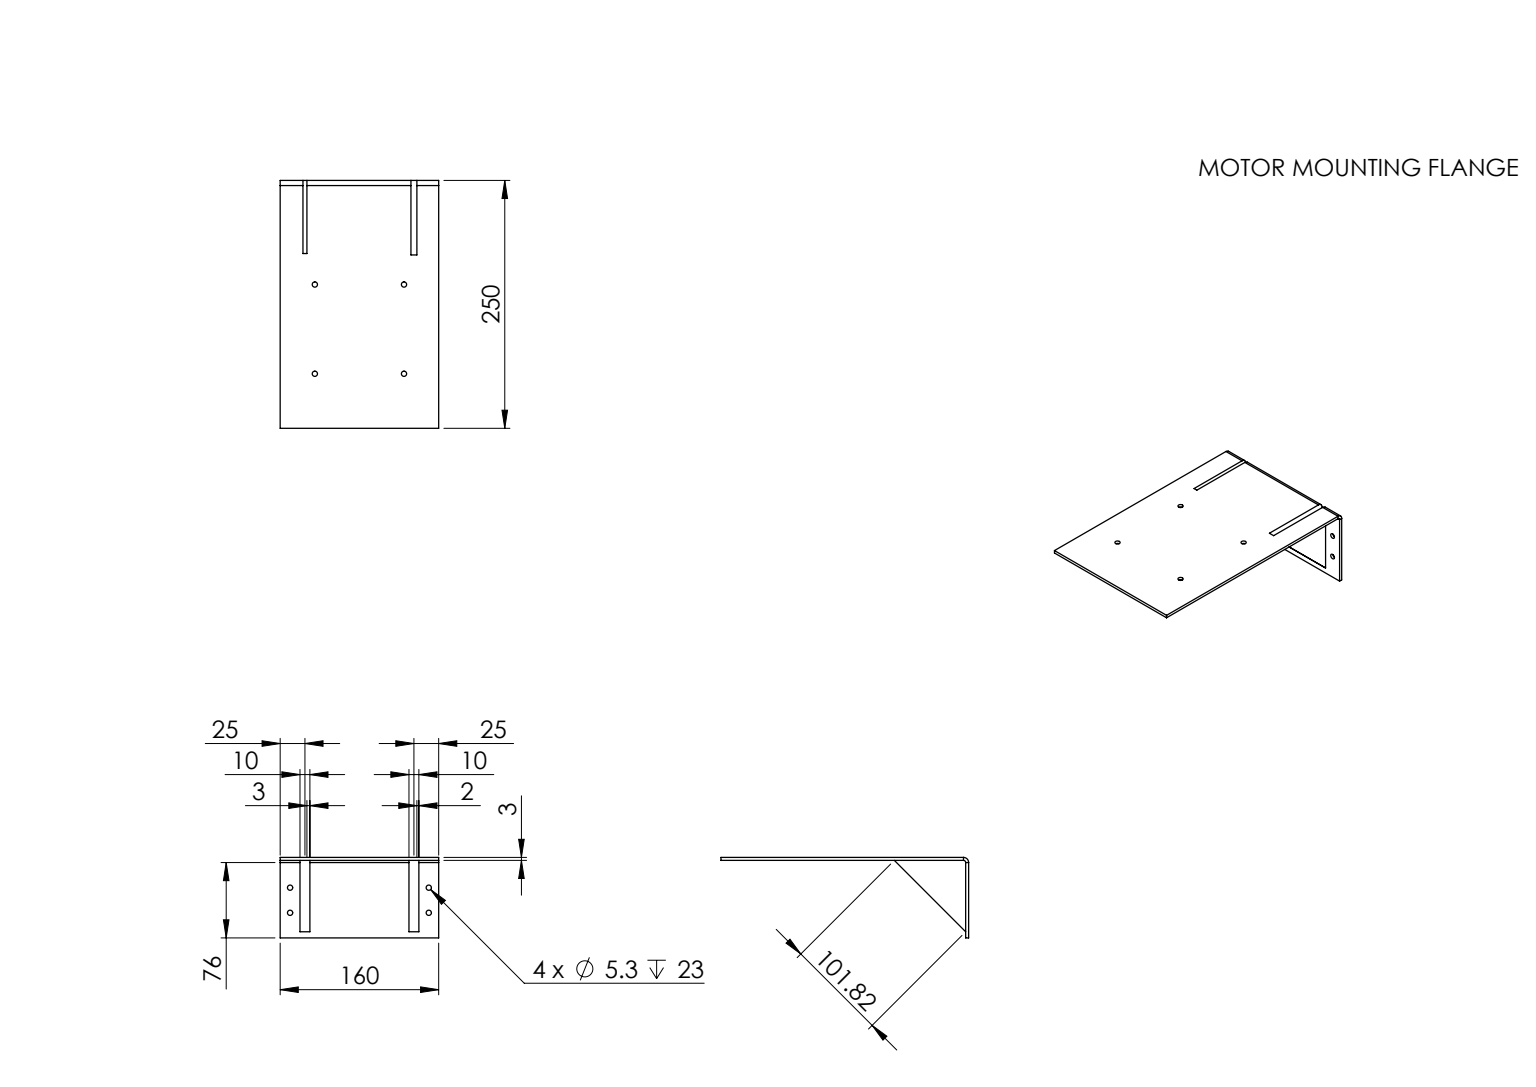
ISO-10303-21;
HEADER;
FILE_DESCRIPTION (('STEP AP214'),
    '1' );
FILE_NAME ('motor mounting flange.step',
    '2026-10-31T03:46:07',
    ( '' ),
    ( '' ),
    'SwSTEP 2.0',
    'SolidWorks 2026',
    '' );
FILE_SCHEMA (( 'AUTOMOTIVE_DESIGN' ));
ENDSEC;

DATA;
#7=VECTOR ( 'NONE', #7349, 1000.000000000000000 ) ;
#29=DIRECTION ( 'NONE',  ( 0.000000000000000000, 0.7071067811865489050, 0.7071067811865462405 ) ) ;
#48=CARTESIAN_POINT ( 'NONE',  ( 80.00000000000004263, -137.9999999999999716, 3.000000000000000000 ) ) ;
#90=EDGE_LOOP ( 'NONE', ( #21123, #7756, #684, #7867 ) ) ;
#122=DIRECTION ( 'NONE',  ( -1.000000000000000000, 3.051161311199799893E-31, 8.144298233840332611E-17 ) ) ;
#142=ORIENTED_EDGE ( 'NONE', *, *, #15816, .T. ) ;
#152=DIRECTION ( 'NONE',  ( 0.000000000000000000, 0.000000000000000000, -1.000000000000000000 ) ) ;
#157=EDGE_CURVE ( 'NONE', #8899, #17134, #9062, .T. ) ;
#169=ORIENTED_EDGE ( 'NONE', *, *, #10857, .T. ) ;
#198=DIRECTION ( 'NONE',  ( 3.469446951953614682E-16, -1.000000000000000000, 3.483493295888648978E-15 ) ) ;
#209=DIRECTION ( 'NONE',  ( 3.469446951953614682E-16, -1.000000000000000000, 3.491481338843133355E-15 ) ) ;
#215=EDGE_CURVE ( 'NONE', #12818, #8899, #13572, .T. ) ;
#237=DIRECTION ( 'NONE',  ( 0.000000000000000000, -1.000000000000000000, 0.000000000000000000 ) ) ;
#240=DIRECTION ( 'NONE',  ( 0.000000000000000000, 0.000000000000000000, -1.000000000000000000 ) ) ;
#241=EDGE_CURVE ( 'NONE', #17193, #16244, #10661, .T. ) ;
#266=ORIENTED_EDGE ( 'NONE', *, *, #12996, .T. ) ;
#269=DIRECTION ( 'NONE',  ( -3.469446951953614682E-16, 1.000000000000000000, -3.483493295888648978E-15 ) ) ;
#281=LINE ( 'NONE', #5839, #17682 ) ;
#317=AXIS2_PLACEMENT_3D ( 'NONE', #22768, #2356, #2723 ) ;
#321=VERTEX_POINT ( 'NONE', #4698 ) ;
#326=VERTEX_POINT ( 'NONE', #2863 ) ;
#327=VERTEX_POINT ( 'NONE', #10267 ) ;
#357=DIRECTION ( 'NONE',  ( 0.000000000000000000, 0.7071067811865485719, 0.7071067811865465735 ) ) ;
#364=DIRECTION ( 'NONE',  ( 0.000000000000000000, -2.618450529776313049E-15, -1.000000000000000000 ) ) ;
#376=AXIS2_PLACEMENT_3D ( 'NONE', #537, #9598, #428 ) ;
#398=AXIS2_PLACEMENT_3D ( 'NONE', #21012, #4473, #22453 ) ;
#403=DIRECTION ( 'NONE',  ( -1.000000000000000000, -0.000000000000000000, -0.000000000000000000 ) ) ;
#428=DIRECTION ( 'NONE',  ( 0.000000000000000000, 1.000000000000000000, -3.502807018799300809E-15 ) ) ;
#444=FACE_BOUND ( 'NONE', #1590, .T. ) ;
#445=DIRECTION ( 'NONE',  ( -0.000000000000000000, -0.000000000000000000, 1.000000000000000000 ) ) ;
#468=ADVANCED_FACE ( 'NONE', ( #22056 ), #1764, .F. ) ;
#506=VERTEX_POINT ( 'NONE', #7097 ) ;
#535=PLANE ( 'NONE',  #3468 ) ;
#537=CARTESIAN_POINT ( 'NONE',  ( -79.99999999999997158, -62.00000000000001421, 5.199999999999997513 ) ) ;
#555=CARTESIAN_POINT ( 'NONE',  ( -69.99999999999997158, -112.6666666666667140, 3.000000000000000000 ) ) ;
#568=DIRECTION ( 'NONE',  ( -1.000000000000000000, -0.000000000000000000, -0.000000000000000000 ) ) ;
#630=CARTESIAN_POINT ( 'NONE',  ( 57.99999999999997868, -62.00000000000001421, -3.122502256758252770E-14 ) ) ;
#633=DIRECTION ( 'NONE',  ( -0.000000000000000000, -0.000000000000000000, 1.000000000000000000 ) ) ;
#644=VERTEX_POINT ( 'NONE', #21439 ) ;
#645=ORIENTED_EDGE ( 'NONE', *, *, #15881, .F. ) ;
#647=EDGE_CURVE ( 'NONE', #8521, #1528, #10238, .T. ) ;
#668=FACE_BOUND ( 'NONE', #1708, .T. ) ;
#684=ORIENTED_EDGE ( 'NONE', *, *, #8782, .F. ) ;
#694=DIRECTION ( 'NONE',  ( 1.000000000000000000, 3.469446951953617640E-16, 8.673617379884035472E-17 ) ) ;
#708=CARTESIAN_POINT ( 'NONE',  ( 45.00000000000004974, -56.79999999999964899, 105.0000000000002132 ) ) ;
#709=VECTOR ( 'NONE', #15669, 1000.000000000000000 ) ;
#741=LINE ( 'NONE', #6187, #22547 ) ;
#743=CIRCLE ( 'NONE', #18865, 2.649999999999985700 ) ;
#789=ORIENTED_EDGE ( 'NONE', *, *, #19625, .F. ) ;
#806=CARTESIAN_POINT ( 'NONE',  ( -69.99999999999997158, -87.33333333333338544, 3.000000000000000000 ) ) ;
#810=CARTESIAN_POINT ( 'NONE',  ( -79.99999999999995737, -62.00000000000004263, 0.000000000000000000 ) ) ;
#814=DIRECTION ( 'NONE',  ( -1.000000000000000000, -3.469446951953613696E-16, 0.000000000000000000 ) ) ;
#824=UNCERTAINTY_MEASURE_WITH_UNIT (LENGTH_MEASURE( 1.000000000000000082E-05 ), #13578, 'distance_accuracy_value', 'NONE');
#832=LINE ( 'NONE', #21116, #18019 ) ;
#837=LINE ( 'NONE', #8216, #5993 ) ;
#848=SURFACE_STYLE_USAGE ( .BOTH. , #23054 ) ;
#849=EDGE_CURVE ( 'NONE', #11269, #12933, #5576, .T. ) ;
#892=ORIENTED_EDGE ( 'NONE', *, *, #1894, .F. ) ;
#897=CARTESIAN_POINT ( 'NONE',  ( 0.000000000000000000, -130.5567675943147492, -0.000000000000000000 ) ) ;
#898=EDGE_CURVE ( 'NONE', #14701, #7954, #741, .T. ) ;
#904=EDGE_CURVE ( 'NONE', #15698, #12205, #4249, .T. ) ;
#912=EDGE_CURVE ( 'NONE', #1785, #23190, #20909, .T. ) ;
#931=VERTEX_POINT ( 'NONE', #630 ) ;
#937=EDGE_CURVE ( 'NONE', #19800, #4863, #16618, .T. ) ;
#958=CIRCLE ( 'NONE', #17951, 2.649999999999999467 ) ;
#959=( LENGTH_UNIT ( ) NAMED_UNIT ( * ) SI_UNIT ( .MILLI., .METRE. ) );
#974=DIRECTION ( 'NONE',  ( -1.000000000000000000, -3.469446951953617640E-16, -8.673617379884035472E-17 ) ) ;
#1008=CYLINDRICAL_SURFACE ( 'NONE', #22278, 2.649999999999985700 ) ;
#1035=ORIENTED_EDGE ( 'NONE', *, *, #13674, .F. ) ;
#1043=FACE_OUTER_BOUND ( 'NONE', #18088, .T. ) ;
#1050=ORIENTED_EDGE ( 'NONE', *, *, #15908, .T. ) ;
#1065=AXIS2_PLACEMENT_3D ( 'NONE', #3394, #1596, #4988 ) ;
#1132=CARTESIAN_POINT ( 'NONE',  ( 52.00000000000000711, -56.80000000000001137, 2.055021403285668792E-13 ) ) ;
#1134=LINE ( 'NONE', #11809, #5012 ) ;
#1166=LINE ( 'NONE', #810, #15749 ) ;
#1170=DIRECTION ( 'NONE',  ( -3.469446951953613696E-16, 1.000000000000000000, 0.000000000000000000 ) ) ;
#1177=CARTESIAN_POINT ( 'NONE',  ( 50.00000000000000000, 0.000000000000000000, 3.000000000000000000 ) ) ;
#1190=EDGE_CURVE ( 'NONE', #13805, #10145, #18337, .T. ) ;
#1192=PLANE ( 'NONE',  #21511 ) ;
#1193=ORIENTED_EDGE ( 'NONE', *, *, #16139, .F. ) ;
#1197=ORIENTED_EDGE ( 'NONE', *, *, #5452, .T. ) ;
#1212=EDGE_CURVE ( 'NONE', #11269, #931, #16668, .T. ) ;
#1214=ORIENTED_EDGE ( 'NONE', *, *, #15943, .F. ) ;
#1222=ORIENTED_EDGE ( 'NONE', *, *, #5330, .T. ) ;
#1225=CARTESIAN_POINT ( 'NONE',  ( 80.00000000000000000, -59.79999999999999005, 3.000000000000000000 ) ) ;
#1247=VERTEX_POINT ( 'NONE', #14867 ) ;
#1266=CARTESIAN_POINT ( 'NONE',  ( -79.99999999999995737, -62.00000000000004263, 0.000000000000000000 ) ) ;
#1275=ORIENTED_EDGE ( 'NONE', *, *, #157, .T. ) ;
#1287=DIRECTION ( 'NONE',  ( 0.000000000000000000, 0.000000000000000000, -1.000000000000000000 ) ) ;
#1310=EDGE_CURVE ( 'NONE', #644, #18250, #10269, .T. ) ;
#1313=ORIENTED_EDGE ( 'NONE', *, *, #647, .F. ) ;
#1315=CYLINDRICAL_SURFACE ( 'NONE', #4216, 2.649999999999999467 ) ;
#1319=AXIS2_PLACEMENT_3D ( 'NONE', #708, #4337, #364 ) ;
#1348=EDGE_LOOP ( 'NONE', ( #12123, #14832, #17782, #8128, #19299, #19905, #4504, #17414, #12961, #17013, #23561, #6301 ) ) ;
#1363=FACE_OUTER_BOUND ( 'NONE', #12024, .T. ) ;
#1374=CARTESIAN_POINT ( 'NONE',  ( 45.00000000000002132, -52.79999999999934346, 195.0000000000002274 ) ) ;
#1422=ORIENTED_EDGE ( 'NONE', *, *, #898, .T. ) ;
#1431=DIRECTION ( 'NONE',  ( -0.000000000000000000, 1.000000000000000000, -3.469446951953613794E-15 ) ) ;
#1438=DIRECTION ( 'NONE',  ( 0.000000000000000000, 2.618450529776326854E-15, 1.000000000000000000 ) ) ;
#1448=ORIENTED_EDGE ( 'NONE', *, *, #7344, .T. ) ;
#1461=VERTEX_POINT ( 'NONE', #6864 ) ;
#1464=EDGE_CURVE ( 'NONE', #10418, #3155, #14145, .T. ) ;
#1465=EDGE_LOOP ( 'NONE', ( #6278, #20700, #142, #6382 ) ) ;
#1471=CARTESIAN_POINT ( 'NONE',  ( -52.99999999999997158, 1.769673560495883054E-29, 4.723692975627390055E-15 ) ) ;
#1475=ORIENTED_EDGE ( 'NONE', *, *, #11144, .F. ) ;
#1482=DIRECTION ( 'NONE',  ( 0.000000000000000000, -0.7071067811865485719, -0.7071067811865465735 ) ) ;
#1494=MECHANICAL_DESIGN_GEOMETRIC_PRESENTATION_REPRESENTATION('',(#21614),#11168);
#1501=ORIENTED_EDGE ( 'NONE', *, *, #13204, .T. ) ;
#1524=VERTEX_POINT ( 'NONE', #12227 ) ;
#1526=CARTESIAN_POINT ( 'NONE',  ( 67.35000000000002274, -87.33333333333332860, 3.000000000000001332 ) ) ;
#1528=VERTEX_POINT ( 'NONE', #10524 ) ;
#1532=FACE_BOUND ( 'NONE', #2193, .T. ) ;
#1589=DIRECTION ( 'NONE',  ( 0.000000000000000000, 1.334402673828305746E-15, -1.000000000000000000 ) ) ;
#1590=EDGE_LOOP ( 'NONE', ( #266, #2447 ) ) ;
#1596=DIRECTION ( 'NONE',  ( -1.000000000000000000, -0.000000000000000000, -0.000000000000000000 ) ) ;
#1598=CARTESIAN_POINT ( 'NONE',  ( -79.99999999999997158, -62.00000000000001421, 5.199999999999997513 ) ) ;
#1600=EDGE_LOOP ( 'NONE', ( #5028, #12753, #23276, #5091 ) ) ;
#1609=ORIENTED_EDGE ( 'NONE', *, *, #2754, .F. ) ;
#1616=CARTESIAN_POINT ( 'NONE',  ( -79.99999999999997158, -62.00000000000001421, 5.199999999999997513 ) ) ;
#1623=CARTESIAN_POINT ( 'NONE',  ( 70.00000000000000000, -112.6666666666666714, 0.000000000000000000 ) ) ;
#1630=ORIENTED_EDGE ( 'NONE', *, *, #4062, .T. ) ;
#1638=CARTESIAN_POINT ( 'NONE',  ( 45.00000000000002132, -56.79999999999933635, 195.0000000000002274 ) ) ;
#1644=CARTESIAN_POINT ( 'NONE',  ( 80.00000000000004263, -137.9999999999999716, 3.000000000000000000 ) ) ;
#1648=ADVANCED_FACE ( 'NONE', ( #21716 ), #5176, .T. ) ;
#1654=DIRECTION ( 'NONE',  ( 0.000000000000000000, 2.618450529776326854E-15, 1.000000000000000000 ) ) ;
#1658=CARTESIAN_POINT ( 'NONE',  ( 80.00000000000004263, -137.9999999999999716, 3.000000000000000000 ) ) ;
#1661=CARTESIAN_POINT ( 'NONE',  ( 52.00000000000000711, 0.000000000000000000, 0.000000000000000000 ) ) ;
#1663=VERTEX_POINT ( 'NONE', #21944 ) ;
#1667=DIRECTION ( 'NONE',  ( 1.000000000000000000, -3.051161311199799893E-31, -8.144298233840332611E-17 ) ) ;
#1681=CARTESIAN_POINT ( 'NONE',  ( -79.99999999999995737, -59.79999999999998295, 5.199999999999989519 ) ) ;
#1684=DIRECTION ( 'NONE',  ( -1.000000000000000000, -3.469446951953614682E-16, -0.000000000000000000 ) ) ;
#1708=EDGE_LOOP ( 'NONE', ( #1630, #19330 ) ) ;
#1709=LINE ( 'NONE', #14329, #18113 ) ;
#1723=ORIENTED_EDGE ( 'NONE', *, *, #14907, .T. ) ;
#1744=ORIENTED_EDGE ( 'NONE', *, *, #6460, .T. ) ;
#1748=DIRECTION ( 'NONE',  ( 1.000000000000000000, 0.000000000000000000, 0.000000000000000000 ) ) ;
#1764=CYLINDRICAL_SURFACE ( 'NONE', #5955, 2.649999999999999467 ) ;
#1783=AXIS2_PLACEMENT_3D ( 'NONE', #13110, #11294, #20425 ) ;
#1785=VERTEX_POINT ( 'NONE', #14685 ) ;
#1796=VERTEX_POINT ( 'NONE', #2374 ) ;
#1797=ADVANCED_FACE ( 'NONE', ( #15318 ), #17117, .T. ) ;
#1799=DIRECTION ( 'NONE',  ( 0.000000000000000000, 1.000000000000000000, -3.502807018799300809E-15 ) ) ;
#1801=CARTESIAN_POINT ( 'NONE',  ( 80.00000000000000000, -61.99999999999998579, 0.000000000000000000 ) ) ;
#1802=ORIENTED_EDGE ( 'NONE', *, *, #11955, .F. ) ;
#1847=CIRCLE ( 'NONE', #22280, 2.200000000000028155 ) ;
#1854=ORIENTED_EDGE ( 'NONE', *, *, #9075, .T. ) ;
#1855=DIRECTION ( 'NONE',  ( 0.000000000000000000, 2.618450529776313049E-15, 1.000000000000000000 ) ) ;
#1884=VECTOR ( 'NONE', #3181, 1000.000000000000000 ) ;
#1888=VECTOR ( 'NONE', #20864, 1000.000000000000000 ) ;
#1894=EDGE_CURVE ( 'NONE', #4011, #20488, #1166, .T. ) ;
#1939=ORIENTED_EDGE ( 'NONE', *, *, #5439, .F. ) ;
#1965=CARTESIAN_POINT ( 'NONE',  ( 80.00000000000001421, -56.79999999999998295, 5.199999999999985967 ) ) ;
#1970=ORIENTED_EDGE ( 'NONE', *, *, #15943, .T. ) ;
#2008=LINE ( 'NONE', #1661, #18975 ) ;
#2014=ORIENTED_EDGE ( 'NONE', *, *, #13472, .F. ) ;
#2017=CARTESIAN_POINT ( 'NONE',  ( -56.99999999999995737, 1.586603881823895016E-29, 4.235035081596970394E-15 ) ) ;
#2027=VERTEX_POINT ( 'NONE', #3439 ) ;
#2051=ORIENTED_EDGE ( 'NONE', *, *, #11144, .T. ) ;
#2099=FACE_BOUND ( 'NONE', #3228, .T. ) ;
#2109=PLANE ( 'NONE',  #11547 ) ;
#2119=CLOSED_SHELL ( 'NONE', ( #11014, #8439, #10072, #10910, #10265, #5080, #12865, #9217, #22299, #4330, #4702, #12929, #9483, #15970, #10638, #16706, #17876, #12809, #18580, #3085, #19020, #1797, #21300, #15713, #21013, #4070, #20526, #23261, #1648, #2484, #22952, #22307, #20455, #20983, #11680, #20762, #3343, #6062, #12723, #11249, #6402, #468, #19361, #22412, #9019, #23041 ) ) ;
#2128=EDGE_LOOP ( 'NONE', ( #13996, #8253, #645, #9491 ) ) ;
#2160=DIRECTION ( 'NONE',  ( -0.000000000000000000, -0.000000000000000000, 1.000000000000000000 ) ) ;
#2193=EDGE_LOOP ( 'NONE', ( #20883, #8607 ) ) ;
#2218=DIRECTION ( 'NONE',  ( -0.000000000000000000, 0.7071067811865485719, 0.7071067811865465735 ) ) ;
#2224=DIRECTION ( 'NONE',  ( -3.469446951953614682E-16, 1.000000000000000000, -3.483493295888648978E-15 ) ) ;
#2255=LINE ( 'NONE', #17249, #15393 ) ;
#2264=AXIS2_PLACEMENT_3D ( 'NONE', #806, #2604, #15082 ) ;
#2280=ORIENTED_EDGE ( 'NONE', *, *, #2696, .F. ) ;
#2296=CARTESIAN_POINT ( 'NONE',  ( 45.00000000000004974, -56.79999999999964899, 105.0000000000002132 ) ) ;
#2334=CARTESIAN_POINT ( 'NONE',  ( 0.000000000000000000, 0.000000000000000000, 3.000000000000000000 ) ) ;
#2356=DIRECTION ( 'NONE',  ( 1.000000000000000000, -0.000000000000000000, 0.000000000000000000 ) ) ;
#2373=EDGE_CURVE ( 'NONE', #12484, #10380, #22971, .T. ) ;
#2374=CARTESIAN_POINT ( 'NONE',  ( -72.64999999999996305, -87.33333333333338544, 0.000000000000000000 ) ) ;
#2405=VERTEX_POINT ( 'NONE', #19951 ) ;
#2417=CARTESIAN_POINT ( 'NONE',  ( -69.99999999999997158, -112.6666666666667140, 3.000000000000001332 ) ) ;
#2423=DIRECTION ( 'NONE',  ( 3.469446951953612710E-16, -1.000000000000000000, 0.000000000000000000 ) ) ;
#2447=ORIENTED_EDGE ( 'NONE', *, *, #16828, .T. ) ;
#2450=CARTESIAN_POINT ( 'NONE',  ( -44.99999999999997868, -59.79999999999937188, 192.3500000000002217 ) ) ;
#2452=DIRECTION ( 'NONE',  ( -3.469446951953614682E-16, 1.000000000000000000, -3.483493295888648978E-15 ) ) ;
#2476=EDGE_CURVE ( 'NONE', #22628, #327, #5234, .T. ) ;
#2484=ADVANCED_FACE ( 'NONE', ( #1363 ), #18035, .F. ) ;
#2486=EDGE_LOOP ( 'NONE', ( #21539, #13879 ) ) ;
#2510=ORIENTED_EDGE ( 'NONE', *, *, #2373, .T. ) ;
#2513=EDGE_CURVE ( 'NONE', #8431, #7697, #1709, .T. ) ;
#2534=DIRECTION ( 'NONE',  ( -0.000000000000000000, 1.000000000000000000, -3.469446951953613794E-15 ) ) ;
#2535=VECTOR ( 'NONE', #1684, 1000.000000000000000 ) ;
#2548=VERTEX_POINT ( 'NONE', #5583 ) ;
#2555=DIRECTION ( 'NONE',  ( 1.211350928885223478E-30, -3.491481338843133355E-15, -1.000000000000000000 ) ) ;
#2591=FACE_OUTER_BOUND ( 'NONE', #2128, .T. ) ;
#2597=CARTESIAN_POINT ( 'NONE',  ( 60.00000000000000000, -59.80000000000001137, 2.159765843450962666E-13 ) ) ;
#2604=DIRECTION ( 'NONE',  ( -0.000000000000000000, -0.000000000000000000, 1.000000000000000000 ) ) ;
#2605=LINE ( 'NONE', #4311, #15382 ) ;
#2629=EDGE_LOOP ( 'NONE', ( #2051, #6281 ) ) ;
#2654=VECTOR ( 'NONE', #23339, 1000.000000000000000 ) ;
#2673=CARTESIAN_POINT ( 'NONE',  ( -67.34999999999996589, -112.6666666666667140, 3.000000000000000000 ) ) ;
#2696=EDGE_CURVE ( 'NONE', #4477, #16291, #13560, .T. ) ;
#2698=AXIS2_PLACEMENT_3D ( 'NONE', #12141, #12505, #19814 ) ;
#2723=DIRECTION ( 'NONE',  ( 0.000000000000000000, 0.000000000000000000, -1.000000000000000000 ) ) ;
#2754=EDGE_CURVE ( 'NONE', #18250, #14819, #6659, .T. ) ;
#2757=DIRECTION ( 'NONE',  ( 3.469446951953614682E-16, -1.000000000000000000, 3.483493295888648978E-15 ) ) ;
#2776=SURFACE_STYLE_FILL_AREA ( #19684 ) ;
#2780=EDGE_CURVE ( 'NONE', #8322, #19974, #4844, .T. ) ;
#2817=LINE ( 'NONE', #22858, #9012 ) ;
#2845=CARTESIAN_POINT ( 'NONE',  ( 67.35000000000002274, -112.6666666666666714, 3.000000000000001332 ) ) ;
#2846=FACE_OUTER_BOUND ( 'NONE', #8329, .T. ) ;
#2862=ORIENTED_EDGE ( 'NONE', *, *, #6325, .T. ) ;
#2863=CARTESIAN_POINT ( 'NONE',  ( -49.99999999999997158, -131.7994082814339833, 3.000000000000017764 ) ) ;
#2887=ORIENTED_EDGE ( 'NONE', *, *, #18974, .F. ) ;
#2917=VERTEX_POINT ( 'NONE', #10012 ) ;
#2925=DIRECTION ( 'NONE',  ( -0.000000000000000000, 3.483493295888648978E-15, 1.000000000000000000 ) ) ;
#2926=ORIENTED_EDGE ( 'NONE', *, *, #17865, .F. ) ;
#2928=FACE_OUTER_BOUND ( 'NONE', #3292, .T. ) ;
#2940=EDGE_CURVE ( 'NONE', #4863, #7697, #8893, .T. ) ;
#2950=AXIS2_PLACEMENT_3D ( 'NONE', #4962, #12382, #16079 ) ;
#2968=VECTOR ( 'NONE', #17545, 1000.000000000000000 ) ;
#2986=DIRECTION ( 'NONE',  ( -0.000000000000000000, -0.000000000000000000, 1.000000000000000000 ) ) ;
#3035=VECTOR ( 'NONE', #22982, 1000.000000000000000 ) ;
#3044=FACE_OUTER_BOUND ( 'NONE', #6003, .T. ) ;
#3068=VECTOR ( 'NONE', #3169, 1000.000000000000000 ) ;
#3079=ORIENTED_EDGE ( 'NONE', *, *, #12259, .T. ) ;
#3085=ADVANCED_FACE ( 'NONE', ( #2846 ), #15915, .T. ) ;
#3155=VERTEX_POINT ( 'NONE', #1526 ) ;
#3169=DIRECTION ( 'NONE',  ( 0.000000000000000000, 3.483493295888648978E-15, 1.000000000000000000 ) ) ;
#3181=DIRECTION ( 'NONE',  ( 5.758888509154132365E-17, 0.7071067811865489050, 0.7071067811865462405 ) ) ;
#3219=CARTESIAN_POINT ( 'NONE',  ( 70.00000000000000000, -87.33333333333332860, 0.000000000000000000 ) ) ;
#3226=ORIENTED_EDGE ( 'NONE', *, *, #17108, .F. ) ;
#3228=EDGE_LOOP ( 'NONE', ( #4081, #20543 ) ) ;
#3230=FACE_BOUND ( 'NONE', #19593, .T. ) ;
#3244=CARTESIAN_POINT ( 'NONE',  ( 59.99999999999998579, -59.79999999999999005, 5.199999999999994849 ) ) ;
#3255=VECTOR ( 'NONE', #2925, 1000.000000000000000 ) ;
#3260=ORIENTED_EDGE ( 'NONE', *, *, #18009, .T. ) ;
#3266=CARTESIAN_POINT ( 'NONE',  ( 0.000000000000000000, -131.9709811566878273, -0.000000000000000000 ) ) ;
#3292=EDGE_LOOP ( 'NONE', ( #5402, #8290, #4208, #23445 ) ) ;
#3320=ORIENTED_EDGE ( 'NONE', *, *, #22824, .T. ) ;
#3330=DIRECTION ( 'NONE',  ( 1.000000000000000000, 0.000000000000000000, 0.000000000000000000 ) ) ;
#3343=ADVANCED_FACE ( 'NONE', ( #3044 ), #8370, .F. ) ;
#3348=DIRECTION ( 'NONE',  ( 0.000000000000000000, 0.000000000000000000, -1.000000000000000000 ) ) ;
#3354=DIRECTION ( 'NONE',  ( -8.144298233840332611E-17, 0.000000000000000000, -1.000000000000000000 ) ) ;
#3357=DIRECTION ( 'NONE',  ( -0.000000000000000000, 1.000000000000000000, -3.469446951953613794E-15 ) ) ;
#3361=DIRECTION ( 'NONE',  ( 1.000000000000000000, 0.000000000000000000, 0.000000000000000000 ) ) ;
#3394=CARTESIAN_POINT ( 'NONE',  ( -79.99999999999995737, -62.00000000000001421, 5.199999999999997513 ) ) ;
#3405=ORIENTED_EDGE ( 'NONE', *, *, #21627, .T. ) ;
#3411=EDGE_LOOP ( 'NONE', ( #1802, #8813 ) ) ;
#3439=CARTESIAN_POINT ( 'NONE',  ( -44.99999999999995026, -59.79999999999969162, 102.3500000000002359 ) ) ;
#3449=DIRECTION ( 'NONE',  ( 0.000000000000000000, 0.000000000000000000, -1.000000000000000000 ) ) ;
#3468=AXIS2_PLACEMENT_3D ( 'NONE', #2334, #22383, #20560 ) ;
#3473=ORIENTED_EDGE ( 'NONE', *, *, #11258, .T. ) ;
#3491=LINE ( 'NONE', #9058, #4168 ) ;
#3508=FACE_OUTER_BOUND ( 'NONE', #3669, .T. ) ;
#3519=DIRECTION ( 'NONE',  ( -0.000000000000000000, -0.000000000000000000, 1.000000000000000000 ) ) ;
#3523=DIRECTION ( 'NONE',  ( 5.478074134663600261E-16, -1.000000000000000000, 0.000000000000000000 ) ) ;
#3530=ORIENTED_EDGE ( 'NONE', *, *, #11258, .F. ) ;
#3535=CARTESIAN_POINT ( 'NONE',  ( 72.64999999999999147, -87.33333333333332860, 3.000000000000000000 ) ) ;
#3570=CARTESIAN_POINT ( 'NONE',  ( -56.99999999999995737, -62.00000000000001421, -3.122502256758252770E-14 ) ) ;
#3577=CARTESIAN_POINT ( 'NONE',  ( -69.99999999999997158, -87.33333333333338544, 0.000000000000000000 ) ) ;
#3610=PLANE ( 'NONE',  #7244 ) ;
#3664=CARTESIAN_POINT ( 'NONE',  ( -44.99999999999995026, -52.79999999999967741, 105.0000000000001990 ) ) ;
#3668=DIRECTION ( 'NONE',  ( -1.000000000000000000, -3.469446951953614682E-16, -0.000000000000000000 ) ) ;
#3669=EDGE_LOOP ( 'NONE', ( #18691, #13001, #20240, #11481 ) ) ;
#3672=DIRECTION ( 'NONE',  ( 3.469446951953614682E-16, -1.000000000000000000, 3.483493295888648978E-15 ) ) ;
#3713=CARTESIAN_POINT ( 'NONE',  ( 70.00000000000000000, -87.33333333333332860, 3.000000000000001332 ) ) ;
#3733=EDGE_CURVE ( 'NONE', #15272, #1785, #17803, .T. ) ;
#3759=VERTEX_POINT ( 'NONE', #22972 ) ;
#3767=DIRECTION ( 'NONE',  ( -0.000000000000000000, -0.000000000000000000, 1.000000000000000000 ) ) ;
#3769=DIRECTION ( 'NONE',  ( 1.000000000000000000, 0.000000000000000000, 0.000000000000000000 ) ) ;
#3799=CARTESIAN_POINT ( 'NONE',  ( 45.00000000000002132, -52.79999999999935056, 192.3500000000002501 ) ) ;
#3819=AXIS2_PLACEMENT_3D ( 'NONE', #2296, #9690, #6285 ) ;
#3822=VECTOR ( 'NONE', #9293, 1000.000000000000000 ) ;
#3844=ORIENTED_EDGE ( 'NONE', *, *, #2754, .T. ) ;
#3910=FACE_OUTER_BOUND ( 'NONE', #7681, .T. ) ;
#3953=PRODUCT_DEFINITION_CONTEXT ( 'detailed design', #14346, 'design' ) ;
#3956=CARTESIAN_POINT ( 'NONE',  ( 60.00000000000000000, 0.000000000000000000, 3.000000000000000000 ) ) ;
#3973=CARTESIAN_POINT ( 'NONE',  ( -79.99999999999994316, -59.79999999999918714, 250.0000000000000000 ) ) ;
#3977=VERTEX_POINT ( 'NONE', #22231 ) ;
#4003=VECTOR ( 'NONE', #3767, 1000.000000000000000 ) ;
#4005=EDGE_CURVE ( 'NONE', #1528, #12933, #5235, .T. ) ;
#4011=VERTEX_POINT ( 'NONE', #13712 ) ;
#4027=DIRECTION ( 'NONE',  ( 1.000000000000000000, 3.469446951953626515E-16, 3.469446951953613203E-16 ) ) ;
#4028=CARTESIAN_POINT ( 'NONE',  ( 0.000000000000000000, 0.000000000000000000, 0.000000000000000000 ) ) ;
#4029=LINE ( 'NONE', #18757, #6734 ) ;
#4062=EDGE_CURVE ( 'NONE', #23038, #15253, #4206, .T. ) ;
#4064=AXIS2_PLACEMENT_3D ( 'NONE', #22627, #11934, #21064 ) ;
#4067=FACE_OUTER_BOUND ( 'NONE', #16357, .T. ) ;
#4070=ADVANCED_FACE ( 'NONE', ( #22365 ), #13238, .F. ) ;
#4074=CARTESIAN_POINT ( 'NONE',  ( -69.99999999999997158, -87.33333333333338544, 0.000000000000000000 ) ) ;
#4080=CARTESIAN_POINT ( 'NONE',  ( 45.00000000000004974, -56.79999999999964189, 107.6500000000002188 ) ) ;
#4081=ORIENTED_EDGE ( 'NONE', *, *, #18682, .F. ) ;
#4094=CARTESIAN_POINT ( 'NONE',  ( 52.00000000000000711, -131.9709811566878273, 2.168404344971008868E-15 ) ) ;
#4127=LINE ( 'NONE', #20196, #19230 ) ;
#4132=EDGE_CURVE ( 'NONE', #4477, #23519, #12032, .T. ) ;
#4136=VECTOR ( 'NONE', #13172, 1000.000000000000000 ) ;
#4159=VECTOR ( 'NONE', #4306, 1000.000000000000000 ) ;
#4168=VECTOR ( 'NONE', #23292, 1000.000000000000000 ) ;
#4172=CARTESIAN_POINT ( 'NONE',  ( 80.00000000000001421, -56.79999999999913030, 250.0000000000000000 ) ) ;
#4206=CIRCLE ( 'NONE', #21171, 2.649999999999985700 ) ;
#4208=ORIENTED_EDGE ( 'NONE', *, *, #21744, .T. ) ;
#4210=CARTESIAN_POINT ( 'NONE',  ( 50.00000000000000000, -131.7994082814339833, 3.000000000000000000 ) ) ;
#4216=AXIS2_PLACEMENT_3D ( 'NONE', #17985, #1431, #16064 ) ;
#4219=AXIS2_PLACEMENT_3D ( 'NONE', #5605, #13013, #18522 ) ;
#4236=ORIENTED_EDGE ( 'NONE', *, *, #18741, .F. ) ;
#4243=VECTOR ( 'NONE', #12870, 1000.000000000000000 ) ;
#4245=CIRCLE ( 'NONE', #13934, 2.200000000000028155 ) ;
#4249=LINE ( 'NONE', #13597, #18307 ) ;
#4285=CARTESIAN_POINT ( 'NONE',  ( 45.00000000000004974, -59.79999999999964899, 105.0000000000002274 ) ) ;
#4297=CYLINDRICAL_SURFACE ( 'NONE', #10029, 2.649999999999999467 ) ;
#4299=DIRECTION ( 'NONE',  ( -3.469446951953612710E-16, 1.000000000000000000, 0.000000000000000000 ) ) ;
#4306=DIRECTION ( 'NONE',  ( 1.000000000000000000, 3.469446951953614189E-16, 0.000000000000000000 ) ) ;
#4311=CARTESIAN_POINT ( 'NONE',  ( -49.99999999999997158, -59.80000000000004690, 2.200487334620165724E-13 ) ) ;
#4330=ADVANCED_FACE ( 'NONE', ( #8836 ), #5318, .T. ) ;
#4337=DIRECTION ( 'NONE',  ( 3.469446951953614682E-16, -1.000000000000000000, 3.483493295888648978E-15 ) ) ;
#4353=EDGE_CURVE ( 'NONE', #12205, #1524, #12617, .T. ) ;
#4397=CARTESIAN_POINT ( 'NONE',  ( -49.99999999999997158, -62.00000000000003553, 3.000000000000000000 ) ) ;
#4413=MANIFOLD_SOLID_BREP ( 'M5 Clearance Hole2', #2119 ) ;
#4418=DIRECTION ( 'NONE',  ( 0.000000000000000000, 2.618450529776326854E-15, 1.000000000000000000 ) ) ;
#4473=DIRECTION ( 'NONE',  ( 3.469446951953614682E-16, -1.000000000000000000, 3.483493295888648978E-15 ) ) ;
#4477=VERTEX_POINT ( 'NONE', #6510 ) ;
#4485=ORIENTED_EDGE ( 'NONE', *, *, #9009, .T. ) ;
#4504=ORIENTED_EDGE ( 'NONE', *, *, #2780, .F. ) ;
#4534=CARTESIAN_POINT ( 'NONE',  ( 70.00000000000000000, -112.6666666666666714, 3.000000000000000000 ) ) ;
#4555=CIRCLE ( 'NONE', #14221, 2.649999999999985700 ) ;
#4566=CARTESIAN_POINT ( 'NONE',  ( -44.99999999999997868, -56.79999999999936477, 195.0000000000001705 ) ) ;
#4575=DIRECTION ( 'NONE',  ( -0.000000000000000000, -0.000000000000000000, -1.000000000000000000 ) ) ;
#4597=CARTESIAN_POINT ( 'NONE',  ( 60.00000000000000000, -59.79999999999974847, 74.99940828143404303 ) ) ;
#4634=EDGE_CURVE ( 'NONE', #327, #7954, #837, .T. ) ;
#4671=CARTESIAN_POINT ( 'NONE',  ( 67.35000000000002274, -87.33333333333332860, 0.000000000000000000 ) ) ;
#4698=CARTESIAN_POINT ( 'NONE',  ( -44.99999999999995026, -56.79999999999967741, 107.6500000000002188 ) ) ;
#4702=ADVANCED_FACE ( 'NONE', ( #14933, #2099, #9493, #3230, #20574 ), #16845, .T. ) ;
#4736=CARTESIAN_POINT ( 'NONE',  ( 1.970645868709624460E-14, -56.79999999999915872, 250.0000000000000000 ) ) ;
#4764=FACE_OUTER_BOUND ( 'NONE', #20383, .T. ) ;
#4798=CARTESIAN_POINT ( 'NONE',  ( -59.99999999999996447, -136.2780879378741474, -5.721320343559392896 ) ) ;
#4805=LINE ( 'NONE', #23022, #21873 ) ;
#4813=ORIENTED_EDGE ( 'NONE', *, *, #14907, .F. ) ;
#4844=LINE ( 'NONE', #7455, #7 ) ;
#4856=CARTESIAN_POINT ( 'NONE',  ( 52.00000000000000711, -62.00000000000001421, 5.199999999999997513 ) ) ;
#4863=VERTEX_POINT ( 'NONE', #13743 ) ;
#4871=EDGE_CURVE ( 'NONE', #18851, #20488, #12999, .T. ) ;
#4936=LINE ( 'NONE', #1658, #14563 ) ;
#4957=PRESENTATION_STYLE_ASSIGNMENT (( #848 ) ) ;
#4962=CARTESIAN_POINT ( 'NONE',  ( -69.99999999999997158, -87.33333333333338544, 3.000000000000001332 ) ) ;
#4970=CARTESIAN_POINT ( 'NONE',  ( -59.99999999999996447, -59.80000000000005400, 2.208631632854006084E-13 ) ) ;
#4980=EDGE_LOOP ( 'NONE', ( #18040, #3405, #18711, #1050 ) ) ;
#4988=DIRECTION ( 'NONE',  ( 0.000000000000000000, 0.000000000000000000, 1.000000000000000000 ) ) ;
#4989=CIRCLE ( 'NONE', #13135, 2.649999999999999467 ) ;
#4996=LINE ( 'NONE', #6319, #12632 ) ;
#4999=EDGE_CURVE ( 'NONE', #23312, #8521, #19360, .T. ) ;
#5011=ADVANCED_BREP_SHAPE_REPRESENTATION ( '', ( #4413, #11210 ), #6181 ) ;
#5012=VECTOR ( 'NONE', #14087, 1000.000000000000000 ) ;
#5028=ORIENTED_EDGE ( 'NONE', *, *, #4871, .F. ) ;
#5031=DIRECTION ( 'NONE',  ( -3.469446951953614682E-16, 1.000000000000000000, -3.483493295888648978E-15 ) ) ;
#5044=ORIENTED_EDGE ( 'NONE', *, *, #21440, .T. ) ;
#5068=VERTEX_POINT ( 'NONE', #12067 ) ;
#5080=ADVANCED_FACE ( 'NONE', ( #2928 ), #12174, .F. ) ;
#5083=ORIENTED_EDGE ( 'NONE', *, *, #14322, .F. ) ;
#5091=ORIENTED_EDGE ( 'NONE', *, *, #1894, .T. ) ;
#5157=PLANE ( 'NONE',  #20763 ) ;
#5170=CIRCLE ( 'NONE', #11755, 2.649999999999999467 ) ;
#5171=ORIENTED_EDGE ( 'NONE', *, *, #18009, .F. ) ;
#5176=PLANE ( 'NONE',  #16406 ) ;
#5189=VECTOR ( 'NONE', #237, 1000.000000000000000 ) ;
#5193=FACE_OUTER_BOUND ( 'NONE', #90, .T. ) ;
#5199=AXIS2_PLACEMENT_3D ( 'NONE', #3664, #14930, #1855 ) ;
#5202=DIRECTION ( 'NONE',  ( 0.000000000000000000, 1.334402673828305746E-15, -1.000000000000000000 ) ) ;
#5204=( GEOMETRIC_REPRESENTATION_CONTEXT ( 3 ) GLOBAL_UNCERTAINTY_ASSIGNED_CONTEXT ( ( #824 ) ) GLOBAL_UNIT_ASSIGNED_CONTEXT ( ( #13578, #13439, #22330 ) ) REPRESENTATION_CONTEXT ( 'NONE', 'WORKASPACE' ) );
#5226=FACE_OUTER_BOUND ( 'NONE', #20922, .T. ) ;
#5227=EDGE_CURVE ( 'NONE', #18517, #6982, #11665, .T. ) ;
#5234=LINE ( 'NONE', #10695, #15031 ) ;
#5235=LINE ( 'NONE', #12641, #12741 ) ;
#5239=EDGE_LOOP ( 'NONE', ( #5299, #10607, #12301, #1609 ) ) ;
#5246=DIRECTION ( 'NONE',  ( -1.000000000000000000, -3.469446951953614682E-16, -0.000000000000000000 ) ) ;
#5255=LINE ( 'NONE', #6957, #23747 ) ;
#5272=CARTESIAN_POINT ( 'NONE',  ( 1.970645868709654753E-14, -56.80000000000003268, 2.055021403285669549E-13 ) ) ;
#5299=ORIENTED_EDGE ( 'NONE', *, *, #16396, .T. ) ;
#5311=AXIS2_PLACEMENT_3D ( 'NONE', #2417, #18954, #17048 ) ;
#5317=ORIENTED_EDGE ( 'NONE', *, *, #11065, .T. ) ;
#5318=CYLINDRICAL_SURFACE ( 'NONE', #16023, 5.200000000000031264 ) ;
#5330=EDGE_CURVE ( 'NONE', #1528, #7205, #6421, .T. ) ;
#5348=VERTEX_POINT ( 'NONE', #19332 ) ;
#5359=PRODUCT ( 'motor mounting flange', 'motor mounting flange', '', ( #14852 ) ) ;
#5394=LINE ( 'NONE', #9377, #11545 ) ;
#5402=ORIENTED_EDGE ( 'NONE', *, *, #18682, .T. ) ;
#5413=CYLINDRICAL_SURFACE ( 'NONE', #17381, 2.649999999999985700 ) ;
#5436=ORIENTED_EDGE ( 'NONE', *, *, #17441, .T. ) ;
#5439=EDGE_CURVE ( 'NONE', #12527, #22261, #23133, .T. ) ;
#5444=ORIENTED_EDGE ( 'NONE', *, *, #4005, .T. ) ;
#5450=FACE_OUTER_BOUND ( 'NONE', #6468, .T. ) ;
#5452=EDGE_CURVE ( 'NONE', #2405, #1528, #17783, .T. ) ;
#5458=ORIENTED_EDGE ( 'NONE', *, *, #12931, .F. ) ;
#5516=DIRECTION ( 'NONE',  ( 1.000000000000000000, 0.000000000000000000, 0.000000000000000000 ) ) ;
#5519=DIRECTION ( 'NONE',  ( 0.000000000000000000, 0.000000000000000000, -1.000000000000000000 ) ) ;
#5527=LINE ( 'NONE', #20362, #8093 ) ;
#5537=CARTESIAN_POINT ( 'NONE',  ( -44.99999999999997868, -59.79999999999935767, 197.6500000000001762 ) ) ;
#5540=VECTOR ( 'NONE', #11579, 1000.000000000000000 ) ;
#5556=LINE ( 'NONE', #20273, #17489 ) ;
#5557=VERTEX_POINT ( 'NONE', #20276 ) ;
#5565=ORIENTED_EDGE ( 'NONE', *, *, #22745, .F. ) ;
#5576=CIRCLE ( 'NONE', #22925, 5.200000000000028599 ) ;
#5583=CARTESIAN_POINT ( 'NONE',  ( -79.99999999999995737, -56.80000000000003979, 5.199999999999971756 ) ) ;
#5590=ORIENTED_EDGE ( 'NONE', *, *, #4005, .F. ) ;
#5605=CARTESIAN_POINT ( 'NONE',  ( -44.99999999999995026, -56.79999999999968452, 105.0000000000002132 ) ) ;
#5722=EDGE_CURVE ( 'NONE', #12103, #321, #9664, .T. ) ;
#5737=CARTESIAN_POINT ( 'NONE',  ( -52.99999999999997158, -56.80000000000003268, 5.199999999999971756 ) ) ;
#5757=CARTESIAN_POINT ( 'NONE',  ( -44.99999999999997868, -52.79999999999936477, 195.0000000000001705 ) ) ;
#5768=AXIS2_PLACEMENT_3D ( 'NONE', #13586, #2534, #15358 ) ;
#5836=ORIENTED_EDGE ( 'NONE', *, *, #4634, .T. ) ;
#5839=CARTESIAN_POINT ( 'NONE',  ( 45.00000000000002132, -52.79999999999933635, 197.6500000000002046 ) ) ;
#5856=LINE ( 'NONE', #8033, #12328 ) ;
#5861=DIRECTION ( 'NONE',  ( 0.000000000000000000, -2.618450529776326854E-15, -1.000000000000000000 ) ) ;
#5889=AXIS2_PLACEMENT_3D ( 'NONE', #3713, #10768, #3361 ) ;
#5916=CARTESIAN_POINT ( 'NONE',  ( 70.00000000000000000, -112.6666666666666714, 3.000000000000000000 ) ) ;
#5951=CARTESIAN_POINT ( 'NONE',  ( -72.64999999999996305, -87.33333333333338544, 3.000000000000000000 ) ) ;
#5955=AXIS2_PLACEMENT_3D ( 'NONE', #10633, #14381, #20241 ) ;
#5978=EDGE_LOOP ( 'NONE', ( #6753, #17830 ) ) ;
#5993=VECTOR ( 'NONE', #13266, 1000.000000000000000 ) ;
#5999=AXIS2_PLACEMENT_3D ( 'NONE', #11082, #3449, #14460 ) ;
#6003=EDGE_LOOP ( 'NONE', ( #12964, #1422, #2014, #19233 ) ) ;
#6044=ORIENTED_EDGE ( 'NONE', *, *, #20262, .F. ) ;
#6062=ADVANCED_FACE ( 'NONE', ( #4067 ), #18565, .T. ) ;
#6078=AXIS2_PLACEMENT_3D ( 'NONE', #7806, #19014, #17226 ) ;
#6081=AXIS2_PLACEMENT_3D ( 'NONE', #16936, #403, #152 ) ;
#6106=CARTESIAN_POINT ( 'NONE',  ( -72.64999999999994884, -87.33333333333338544, 3.000000000000001332 ) ) ;
#6113=CARTESIAN_POINT ( 'NONE',  ( -79.99999999999995737, -138.0000000000000284, 3.000000000000000000 ) ) ;
#6116=ORIENTED_EDGE ( 'NONE', *, *, #22745, .T. ) ;
#6118=CARTESIAN_POINT ( 'NONE',  ( 59.99999999999998579, -62.00000000000001421, 5.199999999999997513 ) ) ;
#6181=( GEOMETRIC_REPRESENTATION_CONTEXT ( 3 ) GLOBAL_UNCERTAINTY_ASSIGNED_CONTEXT ( ( #18338 ) ) GLOBAL_UNIT_ASSIGNED_CONTEXT ( ( #959, #23186, #12017 ) ) REPRESENTATION_CONTEXT ( 'NONE', 'WORKASPACE' ) );
#6187=CARTESIAN_POINT ( 'NONE',  ( -52.99999999999996447, -65.27838379715711881, 65.27838379715736039 ) ) ;
#6257=CARTESIAN_POINT ( 'NONE',  ( 70.00000000000000000, -112.6666666666666714, 3.000000000000001332 ) ) ;
#6278=ORIENTED_EDGE ( 'NONE', *, *, #9712, .F. ) ;
#6281=ORIENTED_EDGE ( 'NONE', *, *, #16521, .T. ) ;
#6285=DIRECTION ( 'NONE',  ( 0.000000000000000000, -2.618450529776313049E-15, -1.000000000000000000 ) ) ;
#6301=ORIENTED_EDGE ( 'NONE', *, *, #10889, .F. ) ;
#6308=EDGE_LOOP ( 'NONE', ( #2280, #5317, #23050, #10213 ) ) ;
#6319=CARTESIAN_POINT ( 'NONE',  ( 80.00000000000001421, -56.79999999999913030, 250.0000000000000000 ) ) ;
#6325=EDGE_CURVE ( 'NONE', #16985, #2548, #10868, .T. ) ;
#6382=ORIENTED_EDGE ( 'NONE', *, *, #5722, .F. ) ;
#6387=ORIENTED_EDGE ( 'NONE', *, *, #12157, .F. ) ;
#6402=ADVANCED_FACE ( 'NONE', ( #11331 ), #4297, .F. ) ;
#6421=LINE ( 'NONE', #15864, #20809 ) ;
#6427=AXIS2_PLACEMENT_3D ( 'NONE', #1598, #17908, #7392 ) ;
#6430=ORIENTED_EDGE ( 'NONE', *, *, #4132, .F. ) ;
#6459=DIRECTION ( 'NONE',  ( -5.618537574013950123E-17, -3.483493295888648978E-15, -1.000000000000000000 ) ) ;
#6460=EDGE_CURVE ( 'NONE', #8431, #19800, #4989, .T. ) ;
#6468=EDGE_LOOP ( 'NONE', ( #6878, #11108, #20530, #2887 ) ) ;
#6469=CIRCLE ( 'NONE', #13835, 2.649999999999985700 ) ;
#6510=CARTESIAN_POINT ( 'NONE',  ( -59.99999999999996447, -59.79999999999998295, 5.199999999999991296 ) ) ;
#6527=( NAMED_UNIT ( * ) SI_UNIT ( $, .STERADIAN. ) SOLID_ANGLE_UNIT ( ) );
#6566=AXIS2_PLACEMENT_3D ( 'NONE', #15094, #22792, #13552 ) ;
#6569=DIRECTION ( 'NONE',  ( 3.469446951953614682E-16, -1.000000000000000000, 3.491481338843133355E-15 ) ) ;
#6572=LINE ( 'NONE', #13735, #2968 ) ;
#6582=CARTESIAN_POINT ( 'NONE',  ( 70.00000000000000000, -87.33333333333332860, 3.000000000000000000 ) ) ;
#6610=CARTESIAN_POINT ( 'NONE',  ( -79.99999999999995737, -62.00000000000004263, 3.000000000000000000 ) ) ;
#6620=DIRECTION ( 'NONE',  ( -0.000000000000000000, 1.000000000000000000, -3.469446951953613794E-15 ) ) ;
#6646=DIRECTION ( 'NONE',  ( -0.000000000000000000, 1.000000000000000000, -3.469446951953613794E-15 ) ) ;
#6657=ORIENTED_EDGE ( 'NONE', *, *, #10573, .T. ) ;
#6659=LINE ( 'NONE', #14057, #21967 ) ;
#6662=ORIENTED_EDGE ( 'NONE', *, *, #19583, .F. ) ;
#6734=VECTOR ( 'NONE', #2218, 1000.000000000000000 ) ;
#6746=DIRECTION ( 'NONE',  ( -0.000000000000000000, -0.000000000000000000, -1.000000000000000000 ) ) ;
#6753=ORIENTED_EDGE ( 'NONE', *, *, #17865, .T. ) ;
#6755=CARTESIAN_POINT ( 'NONE',  ( 45.00000000000004974, -52.79999999999966320, 102.3500000000002075 ) ) ;
#6772=ORIENTED_EDGE ( 'NONE', *, *, #19801, .F. ) ;
#6812=ORIENTED_EDGE ( 'NONE', *, *, #7300, .F. ) ;
#6818=DIRECTION ( 'NONE',  ( -3.469446951953614682E-16, 1.000000000000000000, -3.483493295888648978E-15 ) ) ;
#6834=ORIENTED_EDGE ( 'NONE', *, *, #13697, .T. ) ;
#6845=CYLINDRICAL_SURFACE ( 'NONE', #9815, 2.649999999999985700 ) ;
#6851=ORIENTED_EDGE ( 'NONE', *, *, #2940, .T. ) ;
#6864=CARTESIAN_POINT ( 'NONE',  ( -59.99999999999996447, -131.7994082814339833, 3.000000000000017764 ) ) ;
#6878=ORIENTED_EDGE ( 'NONE', *, *, #19409, .F. ) ;
#6908=CARTESIAN_POINT ( 'NONE',  ( 50.00000000000000000, -59.80000000000001847, 2.159765843450962918E-13 ) ) ;
#6924=FACE_OUTER_BOUND ( 'NONE', #9225, .T. ) ;
#6954=EDGE_CURVE ( 'NONE', #4011, #10831, #2008, .T. ) ;
#6957=CARTESIAN_POINT ( 'NONE',  ( -79.99999999999995737, -56.80000000000006111, 2.099969703877781884E-13 ) ) ;
#6979=DIRECTION ( 'NONE',  ( 0.000000000000000000, 0.7071067811865462405, -0.7071067811865489050 ) ) ;
#6982=VERTEX_POINT ( 'NONE', #7207 ) ;
#6988=ORIENTED_EDGE ( 'NONE', *, *, #11292, .F. ) ;
#6994=ORIENTED_EDGE ( 'NONE', *, *, #1464, .T. ) ;
#6998=DIRECTION ( 'NONE',  ( -1.000000000000000000, 0.000000000000000000, -0.000000000000000000 ) ) ;
#7001=EDGE_LOOP ( 'NONE', ( #6657, #10901 ) ) ;
#7024=DIRECTION ( 'NONE',  ( -1.000000000000000000, 0.000000000000000000, 0.000000000000000000 ) ) ;
#7052=LINE ( 'NONE', #16714, #20006 ) ;
#7061=ORIENTED_EDGE ( 'NONE', *, *, #13329, .F. ) ;
#7062=CYLINDRICAL_SURFACE ( 'NONE', #376, 5.200000000000031264 ) ;
#7097=CARTESIAN_POINT ( 'NONE',  ( 45.00000000000002132, -59.79999999999934346, 192.3500000000002785 ) ) ;
#7137=ORIENTED_EDGE ( 'NONE', *, *, #937, .T. ) ;
#7156=ORIENTED_EDGE ( 'NONE', *, *, #10857, .F. ) ;
#7194=ORIENTED_EDGE ( 'NONE', *, *, #18849, .F. ) ;
#7205=VERTEX_POINT ( 'NONE', #3244 ) ;
#7207=CARTESIAN_POINT ( 'NONE',  ( -49.99999999999997158, -59.79999999999998295, 5.199999999999991296 ) ) ;
#7244=AXIS2_PLACEMENT_3D ( 'NONE', #10555, #16089, #18237 ) ;
#7254=ORIENTED_EDGE ( 'NONE', *, *, #21281, .T. ) ;
#7263=CYLINDRICAL_SURFACE ( 'NONE', #6427, 2.200000000000028155 ) ;
#7267=CIRCLE ( 'NONE', #17684, 5.200000000000028599 ) ;
#7271=AXIS2_PLACEMENT_3D ( 'NONE', #13776, #12321, #14006 ) ;
#7285=CIRCLE ( 'NONE', #20781, 2.649999999999985700 ) ;
#7300=EDGE_CURVE ( 'NONE', #3155, #18160, #16687, .T. ) ;
#7302=CARTESIAN_POINT ( 'NONE',  ( -59.99999999999996447, -62.00000000000001421, 2.999999999999968914 ) ) ;
#7308=VECTOR ( 'NONE', #6459, 1000.000000000000000 ) ;
#7344=EDGE_CURVE ( 'NONE', #5348, #2405, #14397, .T. ) ;
#7349=DIRECTION ( 'NONE',  ( -1.000000000000000000, -3.469446951953627008E-16, -3.469446951953616161E-16 ) ) ;
#7392=DIRECTION ( 'NONE',  ( 0.000000000000000000, 1.000000000000000000, -3.548298019043423769E-15 ) ) ;
#7434=CARTESIAN_POINT ( 'NONE',  ( -69.99999999999997158, -112.6666666666667140, 0.000000000000000000 ) ) ;
#7455=CARTESIAN_POINT ( 'NONE',  ( -5.273354073351990332E-15, -59.79999999999976978, 74.99940828143401461 ) ) ;
#7507=VERTEX_POINT ( 'NONE', #19040 ) ;
#7516=AXIS2_PLACEMENT_3D ( 'NONE', #4028, #23407, #6998 ) ;
#7539=ORIENTED_EDGE ( 'NONE', *, *, #16139, .T. ) ;
#7540=CYLINDRICAL_SURFACE ( 'NONE', #5199, 2.649999999999999467 ) ;
#7542=DIRECTION ( 'NONE',  ( 0.000000000000000000, 0.7071067811865485719, 0.7071067811865465735 ) ) ;
#7566=AXIS2_PLACEMENT_3D ( 'NONE', #18523, #18060, #11073 ) ;
#7582=DIRECTION ( 'NONE',  ( -0.000000000000000000, -0.000000000000000000, 1.000000000000000000 ) ) ;
#7622=ORIENTED_EDGE ( 'NONE', *, *, #5227, .T. ) ;
#7639=ORIENTED_EDGE ( 'NONE', *, *, #22167, .F. ) ;
#7681=EDGE_LOOP ( 'NONE', ( #22011, #10510, #13041, #17510 ) ) ;
#7682=CYLINDRICAL_SURFACE ( 'NONE', #14982, 2.649999999999985700 ) ;
#7687=FACE_OUTER_BOUND ( 'NONE', #17602, .T. ) ;
#7688=DIRECTION ( 'NONE',  ( 0.000000000000000000, -2.838638415234739015E-14, -1.000000000000000000 ) ) ;
#7697=VERTEX_POINT ( 'NONE', #21591 ) ;
#7728=DIRECTION ( 'NONE',  ( -1.000000000000000000, 0.000000000000000000, 0.000000000000000000 ) ) ;
#7735=AXIS2_PLACEMENT_3D ( 'NONE', #2017, #20607, #14972 ) ;
#7756=ORIENTED_EDGE ( 'NONE', *, *, #19801, .T. ) ;
#7761=ORIENTED_EDGE ( 'NONE', *, *, #20262, .T. ) ;
#7765=CARTESIAN_POINT ( 'NONE',  ( -44.99999999999997868, -59.79999999999936477, 195.0000000000001990 ) ) ;
#7793=ORIENTED_EDGE ( 'NONE', *, *, #17108, .T. ) ;
#7795=PLANE ( 'NONE',  #13076 ) ;
#7806=CARTESIAN_POINT ( 'NONE',  ( 70.00000000000000000, -112.6666666666666714, 3.000000000000001332 ) ) ;
#7811=ORIENTED_EDGE ( 'NONE', *, *, #16241, .F. ) ;
#7835=CARTESIAN_POINT ( 'NONE',  ( 72.64999999999999147, -112.6666666666666714, 0.000000000000000000 ) ) ;
#7854=DIRECTION ( 'NONE',  ( 0.000000000000000000, -1.000000000000000000, 0.000000000000000000 ) ) ;
#7867=ORIENTED_EDGE ( 'NONE', *, *, #8713, .F. ) ;
#7897=CARTESIAN_POINT ( 'NONE',  ( 57.99999999999999289, -56.79999999999999005, 5.199999999999971756 ) ) ;
#7913=EDGE_LOOP ( 'NONE', ( #1035, #3473, #9732, #23559 ) ) ;
#7915=CARTESIAN_POINT ( 'NONE',  ( 2.074729277268262863E-14, -59.80000000000003268, 2.159765843450963423E-13 ) ) ;
#7916=DIRECTION ( 'NONE',  ( -1.000000000000000000, 0.000000000000000000, 0.000000000000000000 ) ) ;
#7948=LINE ( 'NONE', #10016, #19983 ) ;
#7954=VERTEX_POINT ( 'NONE', #13873 ) ;
#7986=ORIENTED_EDGE ( 'NONE', *, *, #898, .F. ) ;
#7987=DIRECTION ( 'NONE',  ( 1.000000000000000000, 0.000000000000000000, 0.000000000000000000 ) ) ;
#8017=FACE_BOUND ( 'NONE', #3411, .T. ) ;
#8033=CARTESIAN_POINT ( 'NONE',  ( -5.273354073351953256E-15, -59.79999999999976978, 74.99940828143397198 ) ) ;
#8045=DIRECTION ( 'NONE',  ( 1.000000000000000000, 3.469446951953612710E-16, -5.618537574014070918E-17 ) ) ;
#8055=CARTESIAN_POINT ( 'NONE',  ( -49.99999999999997158, -62.00000000000001421, 5.199999999999997513 ) ) ;
#8093=VECTOR ( 'NONE', #18319, 1000.000000000000000 ) ;
#8128=ORIENTED_EDGE ( 'NONE', *, *, #15980, .F. ) ;
#8129=DIRECTION ( 'NONE',  ( -1.000000000000000000, -3.469446951953627008E-16, -3.469446951953616161E-16 ) ) ;
#8166=FACE_OUTER_BOUND ( 'NONE', #17965, .T. ) ;
#8168=ORIENTED_EDGE ( 'NONE', *, *, #7300, .T. ) ;
#8175=DIRECTION ( 'NONE',  ( 1.000000000000000000, -3.051161311199799893E-31, -8.144298233840332611E-17 ) ) ;
#8183=EDGE_LOOP ( 'NONE', ( #18066, #7254, #20038, #4485, #16729, #23563, #10348, #1275, #22349, #7539, #19190, #14849 ) ) ;
#8199=DIRECTION ( 'NONE',  ( -5.478074134663601247E-16, 1.000000000000000000, 0.000000000000000000 ) ) ;
#8216=CARTESIAN_POINT ( 'NONE',  ( -5.883060564508084174E-15, -56.79999999999977689, 73.75676759431468099 ) ) ;
#8253=ORIENTED_EDGE ( 'NONE', *, *, #10889, .T. ) ;
#8279=CARTESIAN_POINT ( 'NONE',  ( -44.99999999999997868, -56.79999999999935767, 197.6500000000001478 ) ) ;
#8283=CARTESIAN_POINT ( 'NONE',  ( 80.00000000000000000, -56.80000000000000426, 2.010073102693556962E-13 ) ) ;
#8290=ORIENTED_EDGE ( 'NONE', *, *, #2513, .T. ) ;
#8293=CARTESIAN_POINT ( 'NONE',  ( -79.99999999999995737, -62.00000000000004263, 3.000000000000000000 ) ) ;
#8322=VERTEX_POINT ( 'NONE', #4597 ) ;
#8329=EDGE_LOOP ( 'NONE', ( #5590, #1313, #14140, #11197 ) ) ;
#8365=ORIENTED_EDGE ( 'NONE', *, *, #17356, .F. ) ;
#8370=PLANE ( 'NONE',  #15022 ) ;
#8431=VERTEX_POINT ( 'NONE', #8702 ) ;
#8439=ADVANCED_FACE ( 'NONE', ( #5193 ), #19796, .F. ) ;
#8446=ORIENTED_EDGE ( 'NONE', *, *, #13472, .T. ) ;
#8498=ORIENTED_EDGE ( 'NONE', *, *, #912, .T. ) ;
#8521=VERTEX_POINT ( 'NONE', #9416 ) ;
#8575=ORIENTED_EDGE ( 'NONE', *, *, #2373, .F. ) ;
#8607=ORIENTED_EDGE ( 'NONE', *, *, #5439, .T. ) ;
#8608=ORIENTED_EDGE ( 'NONE', *, *, #12694, .T. ) ;
#8625=EDGE_LOOP ( 'NONE', ( #21321, #6812 ) ) ;
#8626=DIRECTION ( 'NONE',  ( 1.000000000000000000, 0.000000000000000000, 0.000000000000000000 ) ) ;
#8637=CARTESIAN_POINT ( 'NONE',  ( 45.00000000000002132, -59.79999999999933635, 195.0000000000002558 ) ) ;
#8644=ORIENTED_EDGE ( 'NONE', *, *, #23781, .T. ) ;
#8651=VECTOR ( 'NONE', #13868, 1000.000000000000000 ) ;
#8657=FACE_OUTER_BOUND ( 'NONE', #21948, .T. ) ;
#8677=VECTOR ( 'NONE', #8129, 1000.000000000000000 ) ;
#8702=CARTESIAN_POINT ( 'NONE',  ( -72.64999999999996305, -112.6666666666667140, 0.000000000000000000 ) ) ;
#8713=EDGE_CURVE ( 'NONE', #23038, #22261, #4805, .T. ) ;
#8716=VECTOR ( 'NONE', #7542, 1000.000000000000000 ) ;
#8724=PLANE ( 'NONE',  #16514 ) ;
#8725=VECTOR ( 'NONE', #10582, 1000.000000000000000 ) ;
#8761=DIRECTION ( 'NONE',  ( 0.000000000000000000, 2.618450529776326854E-15, 1.000000000000000000 ) ) ;
#8782=EDGE_CURVE ( 'NONE', #22261, #12527, #10320, .T. ) ;
#8813=ORIENTED_EDGE ( 'NONE', *, *, #9013, .F. ) ;
#8815=CARTESIAN_POINT ( 'NONE',  ( -59.99999999999996447, -138.3994082814338071, -3.599999999999746070 ) ) ;
#8834=AXIS2_PLACEMENT_3D ( 'NONE', #11819, #8175, #9986 ) ;
#8836=FACE_OUTER_BOUND ( 'NONE', #8873, .T. ) ;
#8858=AXIS2_PLACEMENT_3D ( 'NONE', #15993, #18257, #1482 ) ;
#8873=EDGE_LOOP ( 'NONE', ( #7761, #18869, #20724, #20914 ) ) ;
#8884=CIRCLE ( 'NONE', #13929, 2.649999999999985700 ) ;
#8893=CIRCLE ( 'NONE', #6566, 2.649999999999985700 ) ;
#8899=VERTEX_POINT ( 'NONE', #16288 ) ;
#8922=FACE_BOUND ( 'NONE', #5978, .T. ) ;
#9005=DIRECTION ( 'NONE',  ( 0.000000000000000000, 0.000000000000000000, -1.000000000000000000 ) ) ;
#9009=EDGE_CURVE ( 'NONE', #15698, #23312, #16997, .T. ) ;
#9012=VECTOR ( 'NONE', #17086, 1000.000000000000000 ) ;
#9013=EDGE_CURVE ( 'NONE', #18629, #14819, #10749, .T. ) ;
#9019=ADVANCED_FACE ( 'NONE', ( #20961 ), #7682, .F. ) ;
#9022=PLANE ( 'NONE',  #18269 ) ;
#9023=CARTESIAN_POINT ( 'NONE',  ( 52.00000000000000711, -56.79999999999999005, 5.199999999999971756 ) ) ;
#9058=CARTESIAN_POINT ( 'NONE',  ( -59.99999999999996447, 1.830696786719878692E-29, 3.000000000000000000 ) ) ;
#9060=VERTEX_POINT ( 'NONE', #4172 ) ;
#9062=LINE ( 'NONE', #13078, #21038 ) ;
#9075=EDGE_CURVE ( 'NONE', #7205, #8322, #11586, .T. ) ;
#9078=CARTESIAN_POINT ( 'NONE',  ( -52.99999999999997158, -62.00000000000001421, -3.122502256758252770E-14 ) ) ;
#9083=LINE ( 'NONE', #6908, #17269 ) ;
#9089=CARTESIAN_POINT ( 'NONE',  ( -44.99999999999995026, -52.79999999999968452, 102.3500000000002075 ) ) ;
#9111=EDGE_CURVE ( 'NONE', #10145, #1663, #13876, .T. ) ;
#9112=DIRECTION ( 'NONE',  ( -0.000000000000000000, -0.000000000000000000, 1.000000000000000000 ) ) ;
#9125=CIRCLE ( 'NONE', #2950, 2.649999999999985700 ) ;
#9192=DIRECTION ( 'NONE',  ( 1.000000000000000000, 3.469446951953614189E-16, 0.000000000000000000 ) ) ;
#9217=ADVANCED_FACE ( 'NONE', ( #13994 ), #21319, .F. ) ;
#9225=EDGE_LOOP ( 'NONE', ( #23072, #8365, #21045, #5436 ) ) ;
#9264=CARTESIAN_POINT ( 'NONE',  ( 57.99999999999999289, -135.7851947190609678, -3.814213562373143684 ) ) ;
#9265=CARTESIAN_POINT ( 'NONE',  ( -79.99999999999995737, -62.00000000000004263, 3.000000000000000000 ) ) ;
#9273=EDGE_LOOP ( 'NONE', ( #19309, #21161, #18920, #12618 ) ) ;
#9293=DIRECTION ( 'NONE',  ( -0.000000000000000000, -1.000000000000000000, -0.000000000000000000 ) ) ;
#9315=CARTESIAN_POINT ( 'NONE',  ( -79.99999999999995737, -62.00000000000004263, 0.000000000000000000 ) ) ;
#9356=DIRECTION ( 'NONE',  ( -1.000000000000000000, -0.000000000000000000, -0.000000000000000000 ) ) ;
#9377=CARTESIAN_POINT ( 'NONE',  ( -44.99999999999997868, -52.79999999999937188, 192.3500000000001933 ) ) ;
#9387=ORIENTED_EDGE ( 'NONE', *, *, #23781, .F. ) ;
#9392=LINE ( 'NONE', #14482, #21632 ) ;
#9397=DIRECTION ( 'NONE',  ( 0.000000000000000000, -1.000000000000000000, 0.000000000000000000 ) ) ;
#9414=VECTOR ( 'NONE', #7854, 1000.000000000000000 ) ;
#9416=CARTESIAN_POINT ( 'NONE',  ( 80.00000000000000000, -61.99999999999998579, 3.000000000000000000 ) ) ;
#9467=DIRECTION ( 'NONE',  ( 1.000000000000000000, 3.469446951953617640E-16, 8.673617379884035472E-17 ) ) ;
#9473=CARTESIAN_POINT ( 'NONE',  ( 0.000000000000000000, 0.000000000000000000, 0.000000000000000000 ) ) ;
#9483=ADVANCED_FACE ( 'NONE', ( #15279, #14918, #17196, #8017, #13254 ), #535, .F. ) ;
#9491=ORIENTED_EDGE ( 'NONE', *, *, #16363, .F. ) ;
#9493=FACE_BOUND ( 'NONE', #13465, .T. ) ;
#9494=CIRCLE ( 'NONE', #5999, 2.649999999999999467 ) ;
#9495=CARTESIAN_POINT ( 'NONE',  ( -79.99999999999995737, -62.00000000000001421, 5.199999999999997513 ) ) ;
#9500=CARTESIAN_POINT ( 'NONE',  ( 80.00000000000000000, -56.79999999999998295, 5.199999999999978861 ) ) ;
#9518=CARTESIAN_POINT ( 'NONE',  ( -79.99999999999995737, -138.0000000000000284, 3.000000000000000000 ) ) ;
#9535=AXIS2_PLACEMENT_3D ( 'NONE', #17624, #14043, #1438 ) ;
#9560=VECTOR ( 'NONE', #21605, 1000.000000000000000 ) ;
#9584=EDGE_CURVE ( 'NONE', #18851, #20911, #19106, .T. ) ;
#9598=DIRECTION ( 'NONE',  ( -1.000000000000000000, -0.000000000000000000, -0.000000000000000000 ) ) ;
#9640=DIRECTION ( 'NONE',  ( 0.000000000000000000, 1.000000000000000000, -3.548298019043423769E-15 ) ) ;
#9649=DIRECTION ( 'NONE',  ( -1.000000000000000000, -0.000000000000000000, -0.000000000000000000 ) ) ;
#9664=CIRCLE ( 'NONE', #398, 2.649999999999999467 ) ;
#9668=ORIENTED_EDGE ( 'NONE', *, *, #9584, .F. ) ;
#9669=EDGE_CURVE ( 'NONE', #644, #18629, #12515, .T. ) ;
#9671=DIRECTION ( 'NONE',  ( -1.000000000000000000, 0.000000000000000000, 0.000000000000000000 ) ) ;
#9690=DIRECTION ( 'NONE',  ( 3.469446951953614682E-16, -1.000000000000000000, 3.483493295888648978E-15 ) ) ;
#9712=EDGE_CURVE ( 'NONE', #2027, #12103, #21651, .T. ) ;
#9713=CARTESIAN_POINT ( 'NONE',  ( -56.99999999999995737, -130.5567675943147208, 0.000000000000000000 ) ) ;
#9732=ORIENTED_EDGE ( 'NONE', *, *, #12259, .F. ) ;
#9763=LINE ( 'NONE', #19147, #21172 ) ;
#9801=LINE ( 'NONE', #3973, #20399 ) ;
#9815=AXIS2_PLACEMENT_3D ( 'NONE', #23514, #14369, #1748 ) ;
#9871=DIRECTION ( 'NONE',  ( -1.000000000000000000, 3.051161311199799893E-31, 8.144298233840332611E-17 ) ) ;
#9878=CARTESIAN_POINT ( 'NONE',  ( 80.00000000000000000, -62.00000000000001421, 5.199999999999997513 ) ) ;
#9906=EDGE_CURVE ( 'NONE', #3759, #10418, #8884, .T. ) ;
#9923=EDGE_CURVE ( 'NONE', #10380, #21139, #19669, .T. ) ;
#9948=AXIS2_PLACEMENT_3D ( 'NONE', #3577, #5519, #18425 ) ;
#9964=CIRCLE ( 'NONE', #6081, 2.200000000000028155 ) ;
#9986=DIRECTION ( 'NONE',  ( -8.144298233840332611E-17, 0.000000000000000000, -1.000000000000000000 ) ) ;
#10012=CARTESIAN_POINT ( 'NONE',  ( 57.99999999999999289, -131.9709811566878273, 2.168404344971008868E-15 ) ) ;
#10016=CARTESIAN_POINT ( 'NONE',  ( 80.00000000000001421, -56.79999999999998295, 5.199999999999985967 ) ) ;
#10029=AXIS2_PLACEMENT_3D ( 'NONE', #555, #445, #13390 ) ;
#10072=ADVANCED_FACE ( 'NONE', ( #16048 ), #5413, .F. ) ;
#10103=ORIENTED_EDGE ( 'NONE', *, *, #18741, .T. ) ;
#10107=ORIENTED_EDGE ( 'NONE', *, *, #18465, .F. ) ;
#10145=VERTEX_POINT ( 'NONE', #3570 ) ;
#10150=CARTESIAN_POINT ( 'NONE',  ( 67.35000000000002274, -87.33333333333332860, 3.000000000000000000 ) ) ;
#10176=CARTESIAN_POINT ( 'NONE',  ( -59.99999999999996447, -62.00000000000001421, 5.199999999999997513 ) ) ;
#10213=ORIENTED_EDGE ( 'NONE', *, *, #21281, .F. ) ;
#10238=CIRCLE ( 'NONE', #16393, 2.200000000000028155 ) ;
#10239=DIRECTION ( 'NONE',  ( -1.000000000000000000, -3.469446951953614682E-16, -0.000000000000000000 ) ) ;
#10265=ADVANCED_FACE ( 'NONE', ( #7687 ), #19141, .F. ) ;
#10267=CARTESIAN_POINT ( 'NONE',  ( -56.99999999999995737, -56.79999999999979821, 73.75676759431466678 ) ) ;
#10269=CIRCLE ( 'NONE', #23731, 2.649999999999985700 ) ;
#10270=EDGE_LOOP ( 'NONE', ( #16950, #1744, #7137, #6851 ) ) ;
#10320=CIRCLE ( 'NONE', #18030, 2.649999999999985700 ) ;
#10348=ORIENTED_EDGE ( 'NONE', *, *, #215, .T. ) ;
#10351=CARTESIAN_POINT ( 'NONE',  ( -67.34999999999998010, -87.33333333333338544, 3.000000000000001332 ) ) ;
#10358=EDGE_CURVE ( 'NONE', #13805, #327, #17466, .T. ) ;
#10380=VERTEX_POINT ( 'NONE', #10351 ) ;
#10386=DIRECTION ( 'NONE',  ( -1.000000000000000000, 0.000000000000000000, 0.000000000000000000 ) ) ;
#10418=VERTEX_POINT ( 'NONE', #4671 ) ;
#10499=ORIENTED_EDGE ( 'NONE', *, *, #16521, .F. ) ;
#10510=ORIENTED_EDGE ( 'NONE', *, *, #9712, .T. ) ;
#10524=CARTESIAN_POINT ( 'NONE',  ( 80.00000000000000000, -59.79999999999998295, 5.199999999999989519 ) ) ;
#10528=CARTESIAN_POINT ( 'NONE',  ( -49.99999999999997158, 1.678138721159888895E-29, 4.479364028612180224E-15 ) ) ;
#10555=CARTESIAN_POINT ( 'NONE',  ( 60.00000000000000000, -137.1994082814340743, -2.400000000000046096 ) ) ;
#10573=EDGE_CURVE ( 'NONE', #321, #12103, #23502, .T. ) ;
#10582=DIRECTION ( 'NONE',  ( -5.478074134663601247E-16, 1.000000000000000000, 0.000000000000000000 ) ) ;
#10600=DIRECTION ( 'NONE',  ( 0.000000000000000000, -2.618450529776326854E-15, -1.000000000000000000 ) ) ;
#10607=ORIENTED_EDGE ( 'NONE', *, *, #9669, .T. ) ;
#10630=DIRECTION ( 'NONE',  ( -0.000000000000000000, -0.000000000000000000, 1.000000000000000000 ) ) ;
#10633=CARTESIAN_POINT ( 'NONE',  ( -69.99999999999997158, -87.33333333333338544, 3.000000000000000000 ) ) ;
#10638=ADVANCED_FACE ( 'NONE', ( #16261 ), #7062, .T. ) ;
#10641=ORIENTED_EDGE ( 'NONE', *, *, #13451, .F. ) ;
#10661=CIRCLE ( 'NONE', #1319, 2.649999999999999467 ) ;
#10695=CARTESIAN_POINT ( 'NONE',  ( -56.99999999999995026, -65.27838379715711881, 65.27838379715736039 ) ) ;
#10711=LINE ( 'NONE', #21670, #1884 ) ;
#10738=CARTESIAN_POINT ( 'NONE',  ( 50.00000000000000000, 0.000000000000000000, 0.000000000000000000 ) ) ;
#10745=CARTESIAN_POINT ( 'NONE',  ( 72.64999999999999147, -112.6666666666666714, 3.000000000000001332 ) ) ;
#10749=CIRCLE ( 'NONE', #6078, 2.649999999999985700 ) ;
#10768=DIRECTION ( 'NONE',  ( -0.000000000000000000, -0.000000000000000000, 1.000000000000000000 ) ) ;
#10831=VERTEX_POINT ( 'NONE', #4094 ) ;
#10857=EDGE_CURVE ( 'NONE', #16244, #17193, #20033, .T. ) ;
#10868=LINE ( 'NONE', #12813, #23090 ) ;
#10889=EDGE_CURVE ( 'NONE', #16985, #5348, #9801, .T. ) ;
#10901=ORIENTED_EDGE ( 'NONE', *, *, #5722, .T. ) ;
#10910=ADVANCED_FACE ( 'NONE', ( #22572 ), #18701, .F. ) ;
#10992=ORIENTED_EDGE ( 'NONE', *, *, #9111, .F. ) ;
#11002=FACE_OUTER_BOUND ( 'NONE', #15954, .T. ) ;
#11006=VECTOR ( 'NONE', #3668, 1000.000000000000000 ) ;
#11014=ADVANCED_FACE ( 'NONE', ( #3910 ), #7540, .F. ) ;
#11027=ORIENTED_EDGE ( 'NONE', *, *, #23695, .F. ) ;
#11033=CARTESIAN_POINT ( 'NONE',  ( -56.99999999999995737, -56.80000000000003268, 5.199999999999971756 ) ) ;
#11047=PLANE ( 'NONE',  #21119 ) ;
#11060=DIRECTION ( 'NONE',  ( 8.144298233840332611E-17, 3.483493295888648978E-15, 1.000000000000000000 ) ) ;
#11062=AXIS2_PLACEMENT_3D ( 'NONE', #22495, #2452, #20682 ) ;
#11065=EDGE_CURVE ( 'NONE', #4477, #16985, #2817, .T. ) ;
#11073=DIRECTION ( 'NONE',  ( 0.000000000000000000, -2.618450529776326854E-15, -1.000000000000000000 ) ) ;
#11082=CARTESIAN_POINT ( 'NONE',  ( -69.99999999999997158, -112.6666666666667140, 0.000000000000000000 ) ) ;
#11083=DIRECTION ( 'NONE',  ( 0.000000000000000000, 0.000000000000000000, 1.000000000000000000 ) ) ;
#11108=ORIENTED_EDGE ( 'NONE', *, *, #14124, .T. ) ;
#11113=LINE ( 'NONE', #9518, #3822 ) ;
#11130=VECTOR ( 'NONE', #17819, 1000.000000000000000 ) ;
#11133=UNCERTAINTY_MEASURE_WITH_UNIT (LENGTH_MEASURE( 1.000000000000000082E-05 ), #12242, 'distance_accuracy_value', 'NONE');
#11144=EDGE_CURVE ( 'NONE', #11951, #7507, #14423, .T. ) ;
#11160=VERTEX_POINT ( 'NONE', #4397 ) ;
#11168=( GEOMETRIC_REPRESENTATION_CONTEXT ( 3 ) GLOBAL_UNCERTAINTY_ASSIGNED_CONTEXT ( ( #11133 ) ) GLOBAL_UNIT_ASSIGNED_CONTEXT ( ( #12242, #12376, #6527 ) ) REPRESENTATION_CONTEXT ( 'NONE', 'WORKASPACE' ) );
#11184=VERTEX_POINT ( 'NONE', #19357 ) ;
#11197=ORIENTED_EDGE ( 'NONE', *, *, #849, .T. ) ;
#11210=AXIS2_PLACEMENT_3D ( 'NONE', #9473, #14914, #3769 ) ;
#11249=ADVANCED_FACE ( 'NONE', ( #19594 ), #19470, .F. ) ;
#11258=EDGE_CURVE ( 'NONE', #20911, #23190, #16554, .T. ) ;
#11269=VERTEX_POINT ( 'NONE', #1801 ) ;
#11292=EDGE_CURVE ( 'NONE', #931, #2917, #5556, .T. ) ;
#11294=DIRECTION ( 'NONE',  ( -3.469446951953614682E-16, 1.000000000000000000, -3.483493295888648978E-15 ) ) ;
#11331=FACE_OUTER_BOUND ( 'NONE', #10270, .T. ) ;
#11339=DIRECTION ( 'NONE',  ( 0.000000000000000000, 2.838638415234739015E-14, -1.000000000000000000 ) ) ;
#11340=EDGE_LOOP ( 'NONE', ( #19582, #1475, #15188, #7156 ) ) ;
#11358=CARTESIAN_POINT ( 'NONE',  ( 52.00000000000000711, 0.000000000000000000, 0.000000000000000000 ) ) ;
#11402=ORIENTED_EDGE ( 'NONE', *, *, #16396, .F. ) ;
#11419=LINE ( 'NONE', #1965, #20027 ) ;
#11447=FACE_BOUND ( 'NONE', #2629, .T. ) ;
#11481=ORIENTED_EDGE ( 'NONE', *, *, #157, .F. ) ;
#11484=DIRECTION ( 'NONE',  ( 0.000000000000000000, 0.000000000000000000, -1.000000000000000000 ) ) ;
#11498=ORIENTED_EDGE ( 'NONE', *, *, #16241, .T. ) ;
#11510=EDGE_LOOP ( 'NONE', ( #1222, #1970, #6387, #12828 ) ) ;
#11530=ORIENTED_EDGE ( 'NONE', *, *, #13697, .F. ) ;
#11545=VECTOR ( 'NONE', #18405, 1000.000000000000000 ) ;
#11547=AXIS2_PLACEMENT_3D ( 'NONE', #19008, #8045, #4299 ) ;
#11577=DIRECTION ( 'NONE',  ( 0.000000000000000000, -3.483493295888648978E-15, -1.000000000000000000 ) ) ;
#11579=DIRECTION ( 'NONE',  ( -0.000000000000000000, 1.000000000000000000, -3.469446951953613794E-15 ) ) ;
#11586=LINE ( 'NONE', #2597, #4136 ) ;
#11665=LINE ( 'NONE', #22367, #19899 ) ;
#11680=ADVANCED_FACE ( 'NONE', ( #11002 ), #12710, .T. ) ;
#11710=EDGE_LOOP ( 'NONE', ( #17766, #169 ) ) ;
#11712=CARTESIAN_POINT ( 'NONE',  ( -79.99999999999997158, -62.00000000000001421, 5.199999999999997513 ) ) ;
#11755=AXIS2_PLACEMENT_3D ( 'NONE', #18897, #2224, #22634 ) ;
#11772=CARTESIAN_POINT ( 'NONE',  ( -6.373714457846809652E-15, -56.79999999999976978, 75.17098115668784430 ) ) ;
#11809=CARTESIAN_POINT ( 'NONE',  ( -79.99999999999995737, -138.0000000000000284, 0.000000000000000000 ) ) ;
#11819=CARTESIAN_POINT ( 'NONE',  ( -59.99999999999996447, 1.678138721159888895E-29, 4.479364028612180224E-15 ) ) ;
#11859=LINE ( 'NONE', #14980, #15259 ) ;
#11894=DIRECTION ( 'NONE',  ( 5.758888509154132365E-17, 0.7071067811865489050, 0.7071067811865462405 ) ) ;
#11903=AXIS2_PLACEMENT_3D ( 'NONE', #16587, #20077, #22004 ) ;
#11934=DIRECTION ( 'NONE',  ( -1.000000000000000000, 3.051161311199799893E-31, 8.144298233840332611E-17 ) ) ;
#11937=EDGE_LOOP ( 'NONE', ( #19998, #3320, #21710, #6430 ) ) ;
#11948=DIRECTION ( 'NONE',  ( 1.000000000000000000, 0.000000000000000000, 0.000000000000000000 ) ) ;
#11951=VERTEX_POINT ( 'NONE', #23011 ) ;
#11955=EDGE_CURVE ( 'NONE', #14819, #18629, #15981, .T. ) ;
#12017=( NAMED_UNIT ( * ) SI_UNIT ( $, .STERADIAN. ) SOLID_ANGLE_UNIT ( ) );
#12024=EDGE_LOOP ( 'NONE', ( #20994, #3079, #12986, #4236 ) ) ;
#12032=LINE ( 'NONE', #4970, #21777 ) ;
#12067=CARTESIAN_POINT ( 'NONE',  ( 45.00000000000002132, -59.79999999999933635, 197.6500000000002331 ) ) ;
#12100=FACE_OUTER_BOUND ( 'NONE', #1465, .T. ) ;
#12103=VERTEX_POINT ( 'NONE', #22509 ) ;
#12123=ORIENTED_EDGE ( 'NONE', *, *, #11065, .F. ) ;
#12136=PRODUCT_DEFINITION_SHAPE ( 'NONE', 'NONE',  #17442 ) ;
#12141=CARTESIAN_POINT ( 'NONE',  ( -44.99999999999997868, -56.79999999999936477, 195.0000000000001705 ) ) ;
#12148=EDGE_CURVE ( 'NONE', #2548, #1663, #19055, .T. ) ;
#12157=EDGE_CURVE ( 'NONE', #8521, #12818, #16984, .T. ) ;
#12174=CYLINDRICAL_SURFACE ( 'NONE', #14903, 2.649999999999999467 ) ;
#12205=VERTEX_POINT ( 'NONE', #20217 ) ;
#12227=CARTESIAN_POINT ( 'NONE',  ( 80.00000000000004263, -137.9999999999999716, 0.000000000000000000 ) ) ;
#12242=( LENGTH_UNIT ( ) NAMED_UNIT ( * ) SI_UNIT ( .MILLI., .METRE. ) );
#12256=ORIENTED_EDGE ( 'NONE', *, *, #9669, .F. ) ;
#12259=EDGE_CURVE ( 'NONE', #10831, #23190, #4029, .T. ) ;
#12301=ORIENTED_EDGE ( 'NONE', *, *, #9013, .T. ) ;
#12321=DIRECTION ( 'NONE',  ( 1.000000000000000000, 0.000000000000000000, 0.000000000000000000 ) ) ;
#12328=VECTOR ( 'NONE', #4027, 1000.000000000000000 ) ;
#12361=CARTESIAN_POINT ( 'NONE',  ( 50.00000000000000000, -62.00000000000001421, 2.999999999999968914 ) ) ;
#12376=( NAMED_UNIT ( * ) PLANE_ANGLE_UNIT ( ) SI_UNIT ( $, .RADIAN. ) );
#12382=DIRECTION ( 'NONE',  ( -0.000000000000000000, -0.000000000000000000, 1.000000000000000000 ) ) ;
#12395=CARTESIAN_POINT ( 'NONE',  ( -59.99999999999996447, -138.3994082814338071, -3.599999999999746070 ) ) ;
#12435=DIRECTION ( 'NONE',  ( -0.000000000000000000, -0.000000000000000000, 1.000000000000000000 ) ) ;
#12439=EDGE_LOOP ( 'NONE', ( #15025, #10103, #20613, #6834 ) ) ;
#12465=DIRECTION ( 'NONE',  ( -0.000000000000000000, 1.000000000000000000, -3.469446951953613794E-15 ) ) ;
#12484=VERTEX_POINT ( 'NONE', #13716 ) ;
#12502=CARTESIAN_POINT ( 'NONE',  ( -79.99999999999997158, -62.00000000000001421, 5.199999999999997513 ) ) ;
#12505=DIRECTION ( 'NONE',  ( 3.469446951953614682E-16, -1.000000000000000000, 3.483493295888648978E-15 ) ) ;
#12515=LINE ( 'NONE', #16336, #18127 ) ;
#12523=CARTESIAN_POINT ( 'NONE',  ( -67.34999999999996589, -87.33333333333338544, 3.000000000000000000 ) ) ;
#12527=VERTEX_POINT ( 'NONE', #17307 ) ;
#12585=ORIENTED_EDGE ( 'NONE', *, *, #21744, .F. ) ;
#12586=CARTESIAN_POINT ( 'NONE',  ( 60.00000000000000000, 0.000000000000000000, 0.000000000000000000 ) ) ;
#12602=DIRECTION ( 'NONE',  ( 1.000000000000000000, 3.469446951953614682E-16, -0.000000000000000000 ) ) ;
#12617=LINE ( 'NONE', #18470, #13341 ) ;
#12618=ORIENTED_EDGE ( 'NONE', *, *, #18465, .T. ) ;
#12632=VECTOR ( 'NONE', #6569, 1000.000000000000000 ) ;
#12641=CARTESIAN_POINT ( 'NONE',  ( 80.00000000000000000, -56.79999999999998295, 5.199999999999985967 ) ) ;
#12651=LINE ( 'NONE', #3535, #20593 ) ;
#12694=EDGE_CURVE ( 'NONE', #19415, #17134, #21232, .T. ) ;
#12702=AXIS2_PLACEMENT_3D ( 'NONE', #4798, #6979, #19514 ) ;
#12710=PLANE ( 'NONE',  #20569 ) ;
#12723=ADVANCED_FACE ( 'NONE', ( #1043 ), #13325, .F. ) ;
#12741=VECTOR ( 'NONE', #19952, 1000.000000000000000 ) ;
#12753=ORIENTED_EDGE ( 'NONE', *, *, #9584, .T. ) ;
#12809=ADVANCED_FACE ( 'NONE', ( #16382 ), #9022, .F. ) ;
#12813=CARTESIAN_POINT ( 'NONE',  ( -79.99999999999995737, -59.80000000000003268, 5.199999999999982414 ) ) ;
#12818=VERTEX_POINT ( 'NONE', #23733 ) ;
#12828=ORIENTED_EDGE ( 'NONE', *, *, #647, .T. ) ;
#12864=DIRECTION ( 'NONE',  ( -0.000000000000000000, 3.483493295888648978E-15, 1.000000000000000000 ) ) ;
#12865=ADVANCED_FACE ( 'NONE', ( #16037 ), #6845, .F. ) ;
#12870=DIRECTION ( 'NONE',  ( -0.000000000000000000, 1.000000000000000000, -3.469446951953613794E-15 ) ) ;
#12929=ADVANCED_FACE ( 'NONE', ( #19878, #1532, #8922, #16280, #14466 ), #21807, .F. ) ;
#12931=EDGE_CURVE ( 'NONE', #506, #16172, #20470, .T. ) ;
#12933=VERTEX_POINT ( 'NONE', #9500 ) ;
#12961=ORIENTED_EDGE ( 'NONE', *, *, #5330, .F. ) ;
#12964=ORIENTED_EDGE ( 'NONE', *, *, #17698, .T. ) ;
#12986=ORIENTED_EDGE ( 'NONE', *, *, #912, .F. ) ;
#12996=EDGE_CURVE ( 'NONE', #3977, #2027, #5170, .T. ) ;
#12999=CIRCLE ( 'NONE', #4064, 5.200000000000028599 ) ;
#13001=ORIENTED_EDGE ( 'NONE', *, *, #2780, .T. ) ;
#13013=DIRECTION ( 'NONE',  ( 3.469446951953614682E-16, -1.000000000000000000, 3.483493295888648978E-15 ) ) ;
#13041=ORIENTED_EDGE ( 'NONE', *, *, #10573, .F. ) ;
#13076=AXIS2_PLACEMENT_3D ( 'NONE', #7915, #13747, #11577 ) ;
#13078=CARTESIAN_POINT ( 'NONE',  ( 0.000000000000000000, -131.7994082814339833, 3.000000000000000000 ) ) ;
#13100=ORIENTED_EDGE ( 'NONE', *, *, #9906, .F. ) ;
#13110=CARTESIAN_POINT ( 'NONE',  ( -44.99999999999995026, -59.79999999999968452, 105.0000000000002274 ) ) ;
#13135=AXIS2_PLACEMENT_3D ( 'NONE', #7434, #20703, #7916 ) ;
#13172=DIRECTION ( 'NONE',  ( 0.000000000000000000, 3.483493295888648978E-15, 1.000000000000000000 ) ) ;
#13184=DIRECTION ( 'NONE',  ( 0.000000000000000000, 1.000000000000000000, -3.502807018799300809E-15 ) ) ;
#13204=EDGE_CURVE ( 'NONE', #22628, #14701, #17456, .T. ) ;
#13238=PLANE ( 'NONE',  #16557 ) ;
#13254=FACE_OUTER_BOUND ( 'NONE', #8183, .T. ) ;
#13266=DIRECTION ( 'NONE',  ( 1.000000000000000000, 3.469446951953626515E-16, 3.469446951953613203E-16 ) ) ;
#13280=ORIENTED_EDGE ( 'NONE', *, *, #20532, .F. ) ;
#13300=SHAPE_DEFINITION_REPRESENTATION ( #12136, #19462 ) ;
#13310=ORIENTED_EDGE ( 'NONE', *, *, #1310, .F. ) ;
#13314=DIRECTION ( 'NONE',  ( -1.000000000000000000, 0.000000000000000000, 0.000000000000000000 ) ) ;
#13325=CYLINDRICAL_SURFACE ( 'NONE', #15217, 2.649999999999985700 ) ;
#13329=EDGE_CURVE ( 'NONE', #3759, #18160, #12651, .T. ) ;
#13341=VECTOR ( 'NONE', #9192, 1000.000000000000000 ) ;
#13390=DIRECTION ( 'NONE',  ( 1.000000000000000000, 0.000000000000000000, 0.000000000000000000 ) ) ;
#13403=DIRECTION ( 'NONE',  ( -1.000000000000000000, 0.000000000000000000, -0.000000000000000000 ) ) ;
#13406=EDGE_LOOP ( 'NONE', ( #18963, #12585 ) ) ;
#13439=( NAMED_UNIT ( * ) PLANE_ANGLE_UNIT ( ) SI_UNIT ( $, .RADIAN. ) );
#13448=DIRECTION ( 'NONE',  ( 5.618537574013950123E-17, 3.483493295888648978E-15, 1.000000000000000000 ) ) ;
#13451=EDGE_CURVE ( 'NONE', #1796, #21139, #18382, .T. ) ;
#13465=EDGE_LOOP ( 'NONE', ( #13100, #22217 ) ) ;
#13472=EDGE_CURVE ( 'NONE', #18851, #7954, #4127, .T. ) ;
#13477=AXIS2_PLACEMENT_3D ( 'NONE', #11358, #22544, #18673 ) ;
#13513=LINE ( 'NONE', #22762, #8716 ) ;
#13552=DIRECTION ( 'NONE',  ( 1.000000000000000000, 0.000000000000000000, 0.000000000000000000 ) ) ;
#13560=CIRCLE ( 'NONE', #21976, 2.200000000000028155 ) ;
#13567=ORIENTED_EDGE ( 'NONE', *, *, #2476, .F. ) ;
#13572=LINE ( 'NONE', #3956, #5189 ) ;
#13578=( LENGTH_UNIT ( ) NAMED_UNIT ( * ) SI_UNIT ( .MILLI., .METRE. ) );
#13586=CARTESIAN_POINT ( 'NONE',  ( 45.00000000000004974, -52.79999999999965610, 105.0000000000001990 ) ) ;
#13590=APPLICATION_CONTEXT ( 'automotive_design' ) ;
#13597=CARTESIAN_POINT ( 'NONE',  ( -79.99999999999995737, -138.0000000000000284, 3.000000000000000000 ) ) ;
#13657=CARTESIAN_POINT ( 'NONE',  ( -79.99999999999997158, -62.00000000000001421, 5.199999999999997513 ) ) ;
#13674=EDGE_CURVE ( 'NONE', #20911, #4011, #7267, .T. ) ;
#13689=ORIENTED_EDGE ( 'NONE', *, *, #14394, .F. ) ;
#13696=ORIENTED_EDGE ( 'NONE', *, *, #14394, .T. ) ;
#13697=EDGE_CURVE ( 'NONE', #15272, #931, #17323, .T. ) ;
#13712=CARTESIAN_POINT ( 'NONE',  ( 52.00000000000000711, -62.00000000000001421, -3.122502256758252770E-14 ) ) ;
#13716=CARTESIAN_POINT ( 'NONE',  ( -67.34999999999996589, -87.33333333333338544, 0.000000000000000000 ) ) ;
#13728=DIRECTION ( 'NONE',  ( 1.000000000000000000, 3.469446951953617640E-16, 8.673617379884035472E-17 ) ) ;
#13735=CARTESIAN_POINT ( 'NONE',  ( -52.99999999999997158, 1.617115494935892976E-29, -0.000000000000000000 ) ) ;
#13743=CARTESIAN_POINT ( 'NONE',  ( -67.34999999999998010, -112.6666666666667140, 3.000000000000001332 ) ) ;
#13747=DIRECTION ( 'NONE',  ( 3.469446951953614682E-16, -1.000000000000000000, 3.483493295888648978E-15 ) ) ;
#13772=CARTESIAN_POINT ( 'NONE',  ( -56.99999999999995737, 1.739161947383884814E-29, -0.000000000000000000 ) ) ;
#13776=CARTESIAN_POINT ( 'NONE',  ( 80.00000000000000000, -62.00000000000001421, 5.199999999999997513 ) ) ;
#13805=VERTEX_POINT ( 'NONE', #11033 ) ;
#13819=CARTESIAN_POINT ( 'NONE',  ( 72.64999999999999147, -87.33333333333332860, 3.000000000000001332 ) ) ;
#13820=EDGE_LOOP ( 'NONE', ( #18288, #5836, #7986, #15569 ) ) ;
#13835=AXIS2_PLACEMENT_3D ( 'NONE', #14955, #7582, #5516 ) ;
#13842=CARTESIAN_POINT ( 'NONE',  ( 80.00000000000001421, -56.79999999999998295, 5.199999999999985967 ) ) ;
#13868=DIRECTION ( 'NONE',  ( 1.000000000000000000, 0.000000000000000000, 0.000000000000000000 ) ) ;
#13873=CARTESIAN_POINT ( 'NONE',  ( -52.99999999999996447, -56.79999999999978400, 73.75676759431465257 ) ) ;
#13876=LINE ( 'NONE', #1266, #11130 ) ;
#13879=ORIENTED_EDGE ( 'NONE', *, *, #17663, .F. ) ;
#13880=CARTESIAN_POINT ( 'NONE',  ( -56.99999999999995737, -56.80000000000005400, 2.101443903218560127E-13 ) ) ;
#13893=DIRECTION ( 'NONE',  ( -0.000000000000000000, -0.000000000000000000, -1.000000000000000000 ) ) ;
#13926=VECTOR ( 'NONE', #23411, 1000.000000000000000 ) ;
#13929=AXIS2_PLACEMENT_3D ( 'NONE', #3219, #15931, #10386 ) ;
#13934=AXIS2_PLACEMENT_3D ( 'NONE', #8055, #9871, #11339 ) ;
#13994=FACE_OUTER_BOUND ( 'NONE', #5239, .T. ) ;
#13996=ORIENTED_EDGE ( 'NONE', *, *, #6325, .F. ) ;
#14006=DIRECTION ( 'NONE',  ( 0.000000000000000000, 0.000000000000000000, -1.000000000000000000 ) ) ;
#14043=DIRECTION ( 'NONE',  ( -0.000000000000000000, 1.000000000000000000, -3.469446951953613794E-15 ) ) ;
#14044=SHAPE_REPRESENTATION_RELATIONSHIP ( 'NONE' , 'NONE' ,  #19462, #5011 ) ;
#14057=CARTESIAN_POINT ( 'NONE',  ( 72.64999999999999147, -112.6666666666666714, 3.000000000000000000 ) ) ;
#14066=EDGE_LOOP ( 'NONE', ( #5444, #18000, #17877, #1197 ) ) ;
#14087=DIRECTION ( 'NONE',  ( -0.000000000000000000, -1.000000000000000000, -0.000000000000000000 ) ) ;
#14124=EDGE_CURVE ( 'NONE', #1461, #326, #5527, .T. ) ;
#14127=PLANE ( 'NONE',  #12702 ) ;
#14140=ORIENTED_EDGE ( 'NONE', *, *, #17356, .T. ) ;
#14145=LINE ( 'NONE', #10150, #21019 ) ;
#14212=EDGE_CURVE ( 'NONE', #5557, #15698, #11113, .T. ) ;
#14221=AXIS2_PLACEMENT_3D ( 'NONE', #1638, #3672, #5861 ) ;
#14258=CARTESIAN_POINT ( 'NONE',  ( -79.99999999999995737, -138.0000000000000284, 3.000000000000000000 ) ) ;
#14305=DIRECTION ( 'NONE',  ( 0.000000000000000000, 0.7071067811865462405, -0.7071067811865489050 ) ) ;
#14322=EDGE_CURVE ( 'NONE', #11160, #326, #9763, .T. ) ;
#14329=CARTESIAN_POINT ( 'NONE',  ( -72.64999999999996305, -112.6666666666667140, 3.000000000000000000 ) ) ;
#14330=CARTESIAN_POINT ( 'NONE',  ( 57.99999999999999289, -56.80000000000001137, 2.055021403285668792E-13 ) ) ;
#14332=EDGE_LOOP ( 'NONE', ( #11530, #22656, #22027, #22162 ) ) ;
#14333=ORIENTED_EDGE ( 'NONE', *, *, #241, .F. ) ;
#14346=APPLICATION_CONTEXT ( 'automotive_design' ) ;
#14369=DIRECTION ( 'NONE',  ( -0.000000000000000000, -0.000000000000000000, 1.000000000000000000 ) ) ;
#14381=DIRECTION ( 'NONE',  ( -0.000000000000000000, -0.000000000000000000, 1.000000000000000000 ) ) ;
#14390=LINE ( 'NONE', #8815, #13926 ) ;
#14394=EDGE_CURVE ( 'NONE', #10145, #22628, #15795, .T. ) ;
#14397=LINE ( 'NONE', #18224, #17858 ) ;
#14423=CIRCLE ( 'NONE', #17528, 2.649999999999999467 ) ;
#14432=ORIENTED_EDGE ( 'NONE', *, *, #20078, .F. ) ;
#14460=DIRECTION ( 'NONE',  ( -1.000000000000000000, 0.000000000000000000, 0.000000000000000000 ) ) ;
#14466=FACE_OUTER_BOUND ( 'NONE', #18889, .T. ) ;
#14482=CARTESIAN_POINT ( 'NONE',  ( -79.99999999999995737, -56.79999999999918714, 250.0000000000000000 ) ) ;
#14527=CARTESIAN_POINT ( 'NONE',  ( 70.00000000000000000, -87.33333333333332860, 0.000000000000000000 ) ) ;
#14533=CIRCLE ( 'NONE', #7566, 2.649999999999985700 ) ;
#14542=DIRECTION ( 'NONE',  ( 5.758888509154132365E-17, 0.7071067811865489050, 0.7071067811865462405 ) ) ;
#14554=EDGE_LOOP ( 'NONE', ( #10641, #23102, #2510, #15172 ) ) ;
#14563=VECTOR ( 'NONE', #6746, 1000.000000000000000 ) ;
#14634=AXIS2_PLACEMENT_3D ( 'NONE', #23155, #6620, #15688 ) ;
#14649=DIRECTION ( 'NONE',  ( -1.000000000000000000, 0.000000000000000000, 0.000000000000000000 ) ) ;
#14651=EDGE_LOOP ( 'NONE', ( #10499, #18085, #14333, #14432 ) ) ;
#14683=FACE_OUTER_BOUND ( 'NONE', #11510, .T. ) ;
#14685=CARTESIAN_POINT ( 'NONE',  ( 57.99999999999999289, -56.79999999999974136, 75.17098115668787273 ) ) ;
#14690=ORIENTED_EDGE ( 'NONE', *, *, #1212, .F. ) ;
#14701=VERTEX_POINT ( 'NONE', #20001 ) ;
#14732=ORIENTED_EDGE ( 'NONE', *, *, #1190, .F. ) ;
#14738=FACE_OUTER_BOUND ( 'NONE', #7913, .T. ) ;
#14819=VERTEX_POINT ( 'NONE', #10745 ) ;
#14832=ORIENTED_EDGE ( 'NONE', *, *, #4132, .T. ) ;
#14849=ORIENTED_EDGE ( 'NONE', *, *, #14124, .F. ) ;
#14852=PRODUCT_CONTEXT ( 'NONE', #13590, 'mechanical' ) ;
#14867=CARTESIAN_POINT ( 'NONE',  ( -79.99999999999995737, -56.79999999999918714, 250.0000000000000000 ) ) ;
#14903=AXIS2_PLACEMENT_3D ( 'NONE', #17674, #15893, #23226 ) ;
#14907=EDGE_CURVE ( 'NONE', #6982, #11160, #4245, .T. ) ;
#14913=AXIS2_PLACEMENT_3D ( 'NONE', #1623, #9005, #20101 ) ;
#14914=DIRECTION ( 'NONE',  ( 0.000000000000000000, 0.000000000000000000, 1.000000000000000000 ) ) ;
#14918=FACE_BOUND ( 'NONE', #13406, .T. ) ;
#14930=DIRECTION ( 'NONE',  ( -0.000000000000000000, 1.000000000000000000, -3.469446951953613794E-15 ) ) ;
#14933=FACE_BOUND ( 'NONE', #2486, .T. ) ;
#14941=DIRECTION ( 'NONE',  ( 0.000000000000000000, -3.483493295888648978E-15, -1.000000000000000000 ) ) ;
#14955=CARTESIAN_POINT ( 'NONE',  ( 70.00000000000000000, -87.33333333333332860, 3.000000000000001332 ) ) ;
#14972=DIRECTION ( 'NONE',  ( -8.144298233840332611E-17, 0.000000000000000000, -1.000000000000000000 ) ) ;
#14980=CARTESIAN_POINT ( 'NONE',  ( 50.00000000000000000, -137.1994082814340743, -2.400000000000046096 ) ) ;
#14982=AXIS2_PLACEMENT_3D ( 'NONE', #5757, #20586, #4418 ) ;
#15022=AXIS2_PLACEMENT_3D ( 'NONE', #1471, #21653, #21520 ) ;
#15025=ORIENTED_EDGE ( 'NONE', *, *, #11292, .T. ) ;
#15031=VECTOR ( 'NONE', #14542, 1000.000000000000000 ) ;
#15082=DIRECTION ( 'NONE',  ( 1.000000000000000000, 0.000000000000000000, 0.000000000000000000 ) ) ;
#15083=DIRECTION ( 'NONE',  ( 8.144298233840332611E-17, 3.483493295888648978E-15, 1.000000000000000000 ) ) ;
#15094=CARTESIAN_POINT ( 'NONE',  ( -69.99999999999997158, -112.6666666666667140, 3.000000000000001332 ) ) ;
#15172=ORIENTED_EDGE ( 'NONE', *, *, #9923, .T. ) ;
#15188=ORIENTED_EDGE ( 'NONE', *, *, #20078, .T. ) ;
#15217=AXIS2_PLACEMENT_3D ( 'NONE', #5916, #2160, #20638 ) ;
#15253=VERTEX_POINT ( 'NONE', #2450 ) ;
#15259=VECTOR ( 'NONE', #357, 1000.000000000000000 ) ;
#15272=VERTEX_POINT ( 'NONE', #7897 ) ;
#15279=FACE_BOUND ( 'NONE', #21595, .T. ) ;
#15318=FACE_OUTER_BOUND ( 'NONE', #14332, .T. ) ;
#15353=CARTESIAN_POINT ( 'NONE',  ( -49.99999999999996447, -59.79999999999975557, 74.99940828143398619 ) ) ;
#15358=DIRECTION ( 'NONE',  ( 0.000000000000000000, 2.618450529776313049E-15, 1.000000000000000000 ) ) ;
#15371=DIRECTION ( 'NONE',  ( -0.000000000000000000, -0.000000000000000000, -1.000000000000000000 ) ) ;
#15382=VECTOR ( 'NONE', #15083, 1000.000000000000000 ) ;
#15393=VECTOR ( 'NONE', #8199, 1000.000000000000000 ) ;
#15444=VECTOR ( 'NONE', #13728, 1000.000000000000000 ) ;
#15445=VECTOR ( 'NONE', #16086, 1000.000000000000000 ) ;
#15497=EDGE_LOOP ( 'NONE', ( #22229, #6994, #8168, #7061 ) ) ;
#15503=ORIENTED_EDGE ( 'NONE', *, *, #6954, .T. ) ;
#15547=LINE ( 'NONE', #8283, #7308 ) ;
#15569=ORIENTED_EDGE ( 'NONE', *, *, #13204, .F. ) ;
#15613=DIRECTION ( 'NONE',  ( -0.000000000000000000, -0.000000000000000000, 1.000000000000000000 ) ) ;
#15626=DIRECTION ( 'NONE',  ( 1.000000000000000000, 3.469446951953614682E-16, 0.000000000000000000 ) ) ;
#15634=EDGE_CURVE ( 'NONE', #16985, #5557, #18039, .T. ) ;
#15669=DIRECTION ( 'NONE',  ( -1.000000000000000000, -3.469446951953614682E-16, -0.000000000000000000 ) ) ;
#15688=DIRECTION ( 'NONE',  ( 0.000000000000000000, 2.618450529776313049E-15, 1.000000000000000000 ) ) ;
#15698=VERTEX_POINT ( 'NONE', #14258 ) ;
#15713=ADVANCED_FACE ( 'NONE', ( #20903 ), #1192, .F. ) ;
#15749=VECTOR ( 'NONE', #10239, 1000.000000000000000 ) ;
#15787=DIRECTION ( 'NONE',  ( 1.000000000000000000, 0.000000000000000000, 0.000000000000000000 ) ) ;
#15795=LINE ( 'NONE', #13772, #1888 ) ;
#15797=PLANE ( 'NONE',  #19481 ) ;
#15807=CYLINDRICAL_SURFACE ( 'NONE', #14634, 2.649999999999999467 ) ;
#15816=EDGE_CURVE ( 'NONE', #3977, #321, #18959, .T. ) ;
#15840=FACE_OUTER_BOUND ( 'NONE', #11340, .T. ) ;
#15864=CARTESIAN_POINT ( 'NONE',  ( 80.00000000000001421, -59.79999999999998295, 5.199999999999996625 ) ) ;
#15881=EDGE_CURVE ( 'NONE', #1247, #5348, #9392, .T. ) ;
#15892=CARTESIAN_POINT ( 'NONE',  ( -79.99999999999995737, -62.00000000000001421, 5.199999999999997513 ) ) ;
#15893=DIRECTION ( 'NONE',  ( -0.000000000000000000, -0.000000000000000000, 1.000000000000000000 ) ) ;
#15908=EDGE_CURVE ( 'NONE', #18160, #3155, #6469, .T. ) ;
#15915=PLANE ( 'NONE',  #7271 ) ;
#15931=DIRECTION ( 'NONE',  ( 0.000000000000000000, 0.000000000000000000, -1.000000000000000000 ) ) ;
#15943=EDGE_CURVE ( 'NONE', #7205, #12818, #1847, .T. ) ;
#15954=EDGE_LOOP ( 'NONE', ( #5083, #4813, #21852, #11027 ) ) ;
#15967=DIRECTION ( 'NONE',  ( 8.144298233840332611E-17, 3.483493295888648978E-15, 1.000000000000000000 ) ) ;
#15970=ADVANCED_FACE ( 'NONE', ( #17112 ), #22649, .F. ) ;
#15980=EDGE_CURVE ( 'NONE', #6982, #19241, #2605, .T. ) ;
#15981=CIRCLE ( 'NONE', #17896, 2.649999999999985700 ) ;
#15993=CARTESIAN_POINT ( 'NONE',  ( 60.00000000000000000, -135.7851947190609678, -3.814213562373143684 ) ) ;
#16023=AXIS2_PLACEMENT_3D ( 'NONE', #12502, #23668, #1799 ) ;
#16029=CARTESIAN_POINT ( 'NONE',  ( 50.00000000000000000, -59.79999999999999716, 5.199999999999993960 ) ) ;
#16031=VECTOR ( 'NONE', #13893, 1000.000000000000000 ) ;
#16037=FACE_OUTER_BOUND ( 'NONE', #15497, .T. ) ;
#16048=FACE_OUTER_BOUND ( 'NONE', #18961, .T. ) ;
#16049=CARTESIAN_POINT ( 'NONE',  ( -44.99999999999995026, -52.79999999999967031, 107.6500000000002046 ) ) ;
#16064=DIRECTION ( 'NONE',  ( 0.000000000000000000, 2.618450529776313049E-15, 1.000000000000000000 ) ) ;
#16079=DIRECTION ( 'NONE',  ( 1.000000000000000000, 0.000000000000000000, 0.000000000000000000 ) ) ;
#16086=DIRECTION ( 'NONE',  ( -5.618537574013950123E-17, -3.483493295888648978E-15, -1.000000000000000000 ) ) ;
#16089=DIRECTION ( 'NONE',  ( 0.000000000000000000, -0.7071067811865465735, 0.7071067811865485719 ) ) ;
#16125=AXIS2_PLACEMENT_3D ( 'NONE', #4534, #12435, #11948 ) ;
#16139=EDGE_CURVE ( 'NONE', #19415, #11160, #19616, .T. ) ;
#16169=VECTOR ( 'NONE', #19494, 1000.000000000000000 ) ;
#16172=VERTEX_POINT ( 'NONE', #19378 ) ;
#16224=PRODUCT_DEFINITION_FORMATION_WITH_SPECIFIED_SOURCE ( 'ANY', '', #5359, .NOT_KNOWN. ) ;
#16230=ORIENTED_EDGE ( 'NONE', *, *, #21440, .F. ) ;
#16241=EDGE_CURVE ( 'NONE', #5068, #506, #16897, .T. ) ;
#16244=VERTEX_POINT ( 'NONE', #17941 ) ;
#16261=FACE_OUTER_BOUND ( 'NONE', #1600, .T. ) ;
#16276=CARTESIAN_POINT ( 'NONE',  ( -67.34999999999996589, -112.6666666666667140, 0.000000000000000000 ) ) ;
#16280=FACE_BOUND ( 'NONE', #11710, .T. ) ;
#16288=CARTESIAN_POINT ( 'NONE',  ( 60.00000000000000000, -131.7994082814339833, 3.000000000000000000 ) ) ;
#16291=VERTEX_POINT ( 'NONE', #7302 ) ;
#16292=DIRECTION ( 'NONE',  ( -0.000000000000000000, 1.000000000000000000, -3.469446951953613794E-15 ) ) ;
#16336=CARTESIAN_POINT ( 'NONE',  ( 67.35000000000002274, -112.6666666666666714, 3.000000000000000000 ) ) ;
#16357=EDGE_LOOP ( 'NONE', ( #14732, #18398, #13567, #13689 ) ) ;
#16358=EDGE_CURVE ( 'NONE', #15253, #23038, #14533, .T. ) ;
#16363=EDGE_CURVE ( 'NONE', #2548, #1247, #5255, .T. ) ;
#16382=FACE_OUTER_BOUND ( 'NONE', #9273, .T. ) ;
#16393=AXIS2_PLACEMENT_3D ( 'NONE', #9878, #15787, #17235 ) ;
#16396=EDGE_CURVE ( 'NONE', #18250, #644, #20657, .T. ) ;
#16406=AXIS2_PLACEMENT_3D ( 'NONE', #12586, #19896, #3348 ) ;
#16482=ORIENTED_EDGE ( 'NONE', *, *, #17441, .F. ) ;
#16514=AXIS2_PLACEMENT_3D ( 'NONE', #12395, #14305, #29 ) ;
#16521=EDGE_CURVE ( 'NONE', #7507, #11951, #17989, .T. ) ;
#16554=LINE ( 'NONE', #1132, #3255 ) ;
#16557=AXIS2_PLACEMENT_3D ( 'NONE', #17061, #2555, #18848 ) ;
#16574=EDGE_CURVE ( 'NONE', #9060, #2405, #4996, .T. ) ;
#16587=CARTESIAN_POINT ( 'NONE',  ( 45.00000000000002132, -56.79999999999933635, 195.0000000000002274 ) ) ;
#16618=LINE ( 'NONE', #2673, #21779 ) ;
#16668=LINE ( 'NONE', #9315, #2535 ) ;
#16687=CIRCLE ( 'NONE', #5889, 2.649999999999985700 ) ;
#16706=ADVANCED_FACE ( 'NONE', ( #5226 ), #7263, .F. ) ;
#16714=CARTESIAN_POINT ( 'NONE',  ( -79.99999999999995737, -62.00000000000004263, 3.000000000000000000 ) ) ;
#16729=ORIENTED_EDGE ( 'NONE', *, *, #4999, .T. ) ;
#16735=DIRECTION ( 'NONE',  ( -1.000000000000000000, -0.000000000000000000, -0.000000000000000000 ) ) ;
#16746=ORIENTED_EDGE ( 'NONE', *, *, #15634, .F. ) ;
#16765=AXIS2_PLACEMENT_3D ( 'NONE', #6582, #20159, #8626 ) ;
#16828=EDGE_CURVE ( 'NONE', #2027, #3977, #20290, .T. ) ;
#16845=PLANE ( 'NONE',  #7516 ) ;
#16897=CIRCLE ( 'NONE', #22680, 2.649999999999985700 ) ;
#16933=VECTOR ( 'NONE', #15626, 1000.000000000000000 ) ;
#16936=CARTESIAN_POINT ( 'NONE',  ( 50.00000000000000000, -62.00000000000001421, 5.199999999999997513 ) ) ;
#16950=ORIENTED_EDGE ( 'NONE', *, *, #2513, .F. ) ;
#16984=LINE ( 'NONE', #9265, #11006 ) ;
#16985=VERTEX_POINT ( 'NONE', #1681 ) ;
#16988=FACE_BOUND ( 'NONE', #18199, .T. ) ;
#16997=LINE ( 'NONE', #6113, #4159 ) ;
#17013=ORIENTED_EDGE ( 'NONE', *, *, #5452, .F. ) ;
#17048=DIRECTION ( 'NONE',  ( 1.000000000000000000, 0.000000000000000000, 0.000000000000000000 ) ) ;
#17061=CARTESIAN_POINT ( 'NONE',  ( 80.00000000000001421, -56.79999999999913030, 250.0000000000000000 ) ) ;
#17086=DIRECTION ( 'NONE',  ( -1.000000000000000000, -3.469446951953617640E-16, -8.673617379884035472E-17 ) ) ;
#17108=EDGE_CURVE ( 'NONE', #21139, #10380, #9125, .T. ) ;
#17112=FACE_OUTER_BOUND ( 'NONE', #6308, .T. ) ;
#17117=CYLINDRICAL_SURFACE ( 'NONE', #23454, 5.200000000000031264 ) ;
#17134=VERTEX_POINT ( 'NONE', #4210 ) ;
#17165=CARTESIAN_POINT ( 'NONE',  ( 80.00000000000000000, -56.79999999999999005, 2.999999999999989786 ) ) ;
#17193=VERTEX_POINT ( 'NONE', #4080 ) ;
#17196=FACE_BOUND ( 'NONE', #8625, .T. ) ;
#17226=DIRECTION ( 'NONE',  ( 1.000000000000000000, 0.000000000000000000, 0.000000000000000000 ) ) ;
#17235=DIRECTION ( 'NONE',  ( 0.000000000000000000, 0.000000000000000000, 1.000000000000000000 ) ) ;
#17249=CARTESIAN_POINT ( 'NONE',  ( 80.00000000000004263, -137.9999999999999716, 0.000000000000000000 ) ) ;
#17269=VECTOR ( 'NONE', #12864, 1000.000000000000000 ) ;
#17307=CARTESIAN_POINT ( 'NONE',  ( -44.99999999999997868, -56.79999999999937188, 192.3500000000001933 ) ) ;
#17323=CIRCLE ( 'NONE', #21915, 5.200000000000028599 ) ;
#17356=EDGE_CURVE ( 'NONE', #8521, #11269, #832, .T. ) ;
#17371=DIRECTION ( 'NONE',  ( -3.051161311199799893E-31, -1.000000000000000000, 0.000000000000000000 ) ) ;
#17372=ORIENTED_EDGE ( 'NONE', *, *, #17698, .F. ) ;
#17373=CARTESIAN_POINT ( 'NONE',  ( -79.99999999999995737, -138.0000000000000284, 3.000000000000000000 ) ) ;
#17381=AXIS2_PLACEMENT_3D ( 'NONE', #20349, #16292, #1654 ) ;
#17414=ORIENTED_EDGE ( 'NONE', *, *, #9075, .F. ) ;
#17419=DIRECTION ( 'NONE',  ( -1.000000000000000000, 3.051161311199799893E-31, 8.144298233840332611E-17 ) ) ;
#17441=EDGE_CURVE ( 'NONE', #23312, #1524, #4936, .T. ) ;
#17442=PRODUCT_DEFINITION ( 'UNKNOWN', '', #16224, #3953 ) ;
#17456=LINE ( 'NONE', #897, #8651 ) ;
#17466=LINE ( 'NONE', #13880, #16169 ) ;
#17489=VECTOR ( 'NONE', #17806, 1000.000000000000000 ) ;
#17504=AXIS2_PLACEMENT_3D ( 'NONE', #5272, #198, #14941 ) ;
#17510=ORIENTED_EDGE ( 'NONE', *, *, #15816, .F. ) ;
#17514=ORIENTED_EDGE ( 'NONE', *, *, #904, .T. ) ;
#17528=AXIS2_PLACEMENT_3D ( 'NONE', #4285, #22974, #20941 ) ;
#17545=DIRECTION ( 'NONE',  ( -3.051161311199799893E-31, -1.000000000000000000, 0.000000000000000000 ) ) ;
#17602=EDGE_LOOP ( 'NONE', ( #17859, #20552, #7793, #8575 ) ) ;
#17624=CARTESIAN_POINT ( 'NONE',  ( -44.99999999999997868, -52.79999999999936477, 195.0000000000001705 ) ) ;
#17663=EDGE_CURVE ( 'NONE', #1796, #12484, #18788, .T. ) ;
#17674=CARTESIAN_POINT ( 'NONE',  ( -69.99999999999997158, -112.6666666666667140, 3.000000000000000000 ) ) ;
#17682=VECTOR ( 'NONE', #6646, 1000.000000000000000 ) ;
#17684=AXIS2_PLACEMENT_3D ( 'NONE', #4856, #21859, #19701 ) ;
#17698=EDGE_CURVE ( 'NONE', #20488, #14701, #6572, .T. ) ;
#17726=VECTOR ( 'NONE', #3357, 1000.000000000000000 ) ;
#17766=ORIENTED_EDGE ( 'NONE', *, *, #241, .T. ) ;
#17782=ORIENTED_EDGE ( 'NONE', *, *, #18974, .T. ) ;
#17783=LINE ( 'NONE', #1225, #15445 ) ;
#17803=LINE ( 'NONE', #14330, #3068 ) ;
#17806=DIRECTION ( 'NONE',  ( 0.000000000000000000, -1.000000000000000000, 0.000000000000000000 ) ) ;
#17819=DIRECTION ( 'NONE',  ( -1.000000000000000000, -3.469446951953614682E-16, -0.000000000000000000 ) ) ;
#17825=DIRECTION ( 'NONE',  ( 1.000000000000000000, 0.000000000000000000, 0.000000000000000000 ) ) ;
#17830=ORIENTED_EDGE ( 'NONE', *, *, #22167, .T. ) ;
#17840=DIRECTION ( 'NONE',  ( 1.000000000000000000, 0.000000000000000000, 0.000000000000000000 ) ) ;
#17841=FACE_OUTER_BOUND ( 'NONE', #13820, .T. ) ;
#17858=VECTOR ( 'NONE', #12602, 1000.000000000000000 ) ;
#17859=ORIENTED_EDGE ( 'NONE', *, *, #18331, .T. ) ;
#17865=EDGE_CURVE ( 'NONE', #11184, #16172, #19549, .T. ) ;
#17876=ADVANCED_FACE ( 'NONE', ( #6924 ), #11047, .F. ) ;
#17877=ORIENTED_EDGE ( 'NONE', *, *, #16574, .T. ) ;
#17896=AXIS2_PLACEMENT_3D ( 'NONE', #6257, #19034, #21227 ) ;
#17908=DIRECTION ( 'NONE',  ( -1.000000000000000000, -0.000000000000000000, -0.000000000000000000 ) ) ;
#17925=STYLED_ITEM('',(#23913),#4413);
#17941=CARTESIAN_POINT ( 'NONE',  ( 45.00000000000004974, -56.79999999999965610, 102.3500000000002217 ) ) ;
#17951=AXIS2_PLACEMENT_3D ( 'NONE', #4074, #11484, #9671 ) ;
#17965=EDGE_LOOP ( 'NONE', ( #16746, #2862, #22199, #10107 ) ) ;
#17985=CARTESIAN_POINT ( 'NONE',  ( 45.00000000000004974, -52.79999999999965610, 105.0000000000001990 ) ) ;
#17989=CIRCLE ( 'NONE', #11062, 2.649999999999999467 ) ;
#18000=ORIENTED_EDGE ( 'NONE', *, *, #23579, .F. ) ;
#18009=EDGE_CURVE ( 'NONE', #18517, #19415, #9964, .T. ) ;
#18019=VECTOR ( 'NONE', #4575, 1000.000000000000000 ) ;
#18030=AXIS2_PLACEMENT_3D ( 'NONE', #4566, #2757, #23161 ) ;
#18035=PLANE ( 'NONE',  #8858 ) ;
#18039=CIRCLE ( 'NONE', #1065, 2.200000000000028155 ) ;
#18040=ORIENTED_EDGE ( 'NONE', *, *, #1464, .F. ) ;
#18060=DIRECTION ( 'NONE',  ( -3.469446951953614682E-16, 1.000000000000000000, -3.483493295888648978E-15 ) ) ;
#18066=ORIENTED_EDGE ( 'NONE', *, *, #22824, .F. ) ;
#18078=CARTESIAN_POINT ( 'NONE',  ( -79.99999999999995737, -138.0000000000000284, 3.000000000000000000 ) ) ;
#18080=FACE_OUTER_BOUND ( 'NONE', #18966, .T. ) ;
#18085=ORIENTED_EDGE ( 'NONE', *, *, #19386, .T. ) ;
#18088=EDGE_LOOP ( 'NONE', ( #12256, #19749, #3844, #18326 ) ) ;
#18113=VECTOR ( 'NONE', #21531, 1000.000000000000000 ) ;
#18127=VECTOR ( 'NONE', #3519, 1000.000000000000000 ) ;
#18144=DIRECTION ( 'NONE',  ( 0.000000000000000000, 0.000000000000000000, -1.000000000000000000 ) ) ;
#18160=VERTEX_POINT ( 'NONE', #13819 ) ;
#18181=DIRECTION ( 'NONE',  ( 0.000000000000000000, 0.000000000000000000, 1.000000000000000000 ) ) ;
#18199=EDGE_LOOP ( 'NONE', ( #11498, #8644 ) ) ;
#18224=CARTESIAN_POINT ( 'NONE',  ( 80.00000000000001421, -59.79999999999913030, 250.0000000000000000 ) ) ;
#18237=DIRECTION ( 'NONE',  ( 0.000000000000000000, -0.7071067811865485719, -0.7071067811865465735 ) ) ;
#18250=VERTEX_POINT ( 'NONE', #7835 ) ;
#18257=DIRECTION ( 'NONE',  ( 0.000000000000000000, -0.7071067811865465735, 0.7071067811865485719 ) ) ;
#18269=AXIS2_PLACEMENT_3D ( 'NONE', #18078, #17840, #1287 ) ;
#18278=EDGE_CURVE ( 'NONE', #17134, #19974, #11859, .T. ) ;
#18281=AXIS2_PLACEMENT_3D ( 'NONE', #9495, #16735, #11083 ) ;
#18288=ORIENTED_EDGE ( 'NONE', *, *, #2476, .T. ) ;
#18289=DIRECTION ( 'NONE',  ( 0.000000000000000000, 0.7071067811865485719, 0.7071067811865465735 ) ) ;
#18307=VECTOR ( 'NONE', #15371, 1000.000000000000000 ) ;
#18319=DIRECTION ( 'NONE',  ( 1.000000000000000000, 0.000000000000000000, 0.000000000000000000 ) ) ;
#18326=ORIENTED_EDGE ( 'NONE', *, *, #11955, .T. ) ;
#18331=EDGE_CURVE ( 'NONE', #12484, #1796, #958, .T. ) ;
#18337=CIRCLE ( 'NONE', #23360, 5.200000000000028599 ) ;
#18338=UNCERTAINTY_MEASURE_WITH_UNIT (LENGTH_MEASURE( 1.000000000000000082E-05 ), #959, 'distance_accuracy_value', 'NONE');
#18382=LINE ( 'NONE', #5951, #4003 ) ;
#18398=ORIENTED_EDGE ( 'NONE', *, *, #10358, .T. ) ;
#18405=DIRECTION ( 'NONE',  ( -0.000000000000000000, 1.000000000000000000, -3.469446951953613794E-15 ) ) ;
#18425=DIRECTION ( 'NONE',  ( -1.000000000000000000, 0.000000000000000000, 0.000000000000000000 ) ) ;
#18465=EDGE_CURVE ( 'NONE', #5557, #1663, #21578, .T. ) ;
#18470=CARTESIAN_POINT ( 'NONE',  ( -79.99999999999995737, -138.0000000000000284, 0.000000000000000000 ) ) ;
#18517=VERTEX_POINT ( 'NONE', #16029 ) ;
#18522=DIRECTION ( 'NONE',  ( 0.000000000000000000, -2.618450529776313049E-15, -1.000000000000000000 ) ) ;
#18523=CARTESIAN_POINT ( 'NONE',  ( -44.99999999999997868, -59.79999999999936477, 195.0000000000001990 ) ) ;
#18565=PLANE ( 'NONE',  #7735 ) ;
#18580=ADVANCED_FACE ( 'NONE', ( #8657 ), #15797, .F. ) ;
#18629=VERTEX_POINT ( 'NONE', #2845 ) ;
#18666=ORIENTED_EDGE ( 'NONE', *, *, #23579, .T. ) ;
#18673=DIRECTION ( 'NONE',  ( 0.000000000000000000, 0.000000000000000000, -1.000000000000000000 ) ) ;
#18682=EDGE_CURVE ( 'NONE', #19800, #8431, #9494, .T. ) ;
#18691=ORIENTED_EDGE ( 'NONE', *, *, #18849, .T. ) ;
#18701=CYLINDRICAL_SURFACE ( 'NONE', #5768, 2.649999999999999467 ) ;
#18711=ORIENTED_EDGE ( 'NONE', *, *, #13329, .T. ) ;
#18741=EDGE_CURVE ( 'NONE', #2917, #1785, #23724, .T. ) ;
#18757=CARTESIAN_POINT ( 'NONE',  ( 52.00000000000000711, -135.7851947190609678, -3.814213562373143684 ) ) ;
#18788=CIRCLE ( 'NONE', #9948, 2.649999999999999467 ) ;
#18848=DIRECTION ( 'NONE',  ( 0.000000000000000000, 1.000000000000000000, -3.491481338843133355E-15 ) ) ;
#18849=EDGE_CURVE ( 'NONE', #8899, #8322, #13513, .T. ) ;
#18851=VERTEX_POINT ( 'NONE', #5737 ) ;
#18865=AXIS2_PLACEMENT_3D ( 'NONE', #8637, #6818, #21550 ) ;
#18869=ORIENTED_EDGE ( 'NONE', *, *, #1190, .T. ) ;
#18889=EDGE_LOOP ( 'NONE', ( #21002, #6044, #20187, #5044, #18666, #6662, #21626, #8498, #3530, #9668, #8446, #20494 ) ) ;
#18894=PLANE ( 'NONE',  #317 ) ;
#18897=CARTESIAN_POINT ( 'NONE',  ( -44.99999999999995026, -59.79999999999968452, 105.0000000000002274 ) ) ;
#18898=PLANE ( 'NONE',  #8834 ) ;
#18920=ORIENTED_EDGE ( 'NONE', *, *, #14212, .F. ) ;
#18940=CARTESIAN_POINT ( 'NONE',  ( 70.00000000000000000, -112.6666666666666714, 0.000000000000000000 ) ) ;
#18954=DIRECTION ( 'NONE',  ( -0.000000000000000000, -0.000000000000000000, 1.000000000000000000 ) ) ;
#18959=LINE ( 'NONE', #16049, #9560 ) ;
#18961=EDGE_LOOP ( 'NONE', ( #9387, #19100, #2926, #5565 ) ) ;
#18963=ORIENTED_EDGE ( 'NONE', *, *, #2940, .F. ) ;
#18966=EDGE_LOOP ( 'NONE', ( #22188, #3260, #8608, #23374 ) ) ;
#18967=DIRECTION ( 'NONE',  ( 0.000000000000000000, 0.000000000000000000, -1.000000000000000000 ) ) ;
#18974=EDGE_CURVE ( 'NONE', #23519, #19241, #5856, .T. ) ;
#18975=VECTOR ( 'NONE', #9397, 1000.000000000000000 ) ;
#19008=CARTESIAN_POINT ( 'NONE',  ( -79.99999999999994316, -56.79999999999918714, 250.0000000000000000 ) ) ;
#19013=EDGE_CURVE ( 'NONE', #1663, #12205, #1134, .T. ) ;
#19014=DIRECTION ( 'NONE',  ( -0.000000000000000000, -0.000000000000000000, 1.000000000000000000 ) ) ;
#19020=ADVANCED_FACE ( 'NONE', ( #8166 ), #21187, .F. ) ;
#19034=DIRECTION ( 'NONE',  ( -0.000000000000000000, -0.000000000000000000, 1.000000000000000000 ) ) ;
#19040=CARTESIAN_POINT ( 'NONE',  ( 45.00000000000004974, -59.79999999999965610, 102.3500000000002359 ) ) ;
#19055=CIRCLE ( 'NONE', #18281, 5.200000000000028599 ) ;
#19065=MECHANICAL_DESIGN_GEOMETRIC_PRESENTATION_REPRESENTATION('',(#17925),#5204);
#19100=ORIENTED_EDGE ( 'NONE', *, *, #12931, .T. ) ;
#19106=LINE ( 'NONE', #13842, #15444 ) ;
#19122=DIRECTION ( 'NONE',  ( 0.000000000000000000, 0.000000000000000000, -1.000000000000000000 ) ) ;
#19141=CYLINDRICAL_SURFACE ( 'NONE', #2264, 2.649999999999999467 ) ;
#19147=CARTESIAN_POINT ( 'NONE',  ( -49.99999999999997158, 1.525580655599899097E-29, 3.000000000000000000 ) ) ;
#19190=ORIENTED_EDGE ( 'NONE', *, *, #14322, .T. ) ;
#19209=AXIS2_PLACEMENT_3D ( 'NONE', #11712, #568, #9640 ) ;
#19230=VECTOR ( 'NONE', #11060, 1000.000000000000000 ) ;
#19233=ORIENTED_EDGE ( 'NONE', *, *, #4871, .T. ) ;
#19241=VERTEX_POINT ( 'NONE', #15353 ) ;
#19252=CARTESIAN_POINT ( 'NONE',  ( 45.00000000000004974, -52.79999999999964899, 107.6500000000002046 ) ) ;
#19254=FACE_OUTER_BOUND ( 'NONE', #12439, .T. ) ;
#19299=ORIENTED_EDGE ( 'NONE', *, *, #5227, .F. ) ;
#19309=ORIENTED_EDGE ( 'NONE', *, *, #19013, .T. ) ;
#19318=FILL_AREA_STYLE_COLOUR ( '', #19667 ) ;
#19330=ORIENTED_EDGE ( 'NONE', *, *, #16358, .T. ) ;
#19332=CARTESIAN_POINT ( 'NONE',  ( -79.99999999999995737, -59.79999999999918714, 250.0000000000000000 ) ) ;
#19357=CARTESIAN_POINT ( 'NONE',  ( 45.00000000000002132, -56.79999999999932925, 197.6500000000002046 ) ) ;
#19360=LINE ( 'NONE', #21663, #8725 ) ;
#19361=ADVANCED_FACE ( 'NONE', ( #15840 ), #1315, .F. ) ;
#19378=CARTESIAN_POINT ( 'NONE',  ( 45.00000000000002132, -56.79999999999934346, 192.3500000000002501 ) ) ;
#19386=EDGE_CURVE ( 'NONE', #7507, #16244, #23175, .T. ) ;
#19409=EDGE_CURVE ( 'NONE', #1461, #23519, #14390, .T. ) ;
#19415=VERTEX_POINT ( 'NONE', #12361 ) ;
#19435=ORIENTED_EDGE ( 'NONE', *, *, #4353, .T. ) ;
#19462=SHAPE_REPRESENTATION ( 'motor mounting flange', ( #11210 ), #6181 ) ;
#19470=CYLINDRICAL_SURFACE ( 'NONE', #16765, 2.649999999999985700 ) ;
#19476=LINE ( 'NONE', #19252, #3035 ) ;
#19481=AXIS2_PLACEMENT_3D ( 'NONE', #17373, #1170, #814 ) ;
#19494=DIRECTION ( 'NONE',  ( 8.144298233840332611E-17, 3.483493295888648978E-15, 1.000000000000000000 ) ) ;
#19514=DIRECTION ( 'NONE',  ( 0.000000000000000000, 0.7071067811865489050, 0.7071067811865462405 ) ) ;
#19549=CIRCLE ( 'NONE', #11903, 2.649999999999985700 ) ;
#19568=LINE ( 'NONE', #4736, #16933 ) ;
#19582=ORIENTED_EDGE ( 'NONE', *, *, #19386, .F. ) ;
#19583=EDGE_CURVE ( 'NONE', #15272, #12933, #7948, .T. ) ;
#19593=EDGE_LOOP ( 'NONE', ( #11402, #13310 ) ) ;
#19594=FACE_OUTER_BOUND ( 'NONE', #4980, .T. ) ;
#19616=LINE ( 'NONE', #8293, #709 ) ;
#19625=EDGE_CURVE ( 'NONE', #1524, #11269, #2255, .T. ) ;
#19667=COLOUR_RGB ( '',0.8941176470588234615, 0.8941176470588234615, 0.8941176470588234615 ) ;
#19669=CIRCLE ( 'NONE', #23132, 2.649999999999985700 ) ;
#19684=FILL_AREA_STYLE ('',( #19318 ) ) ;
#19701=DIRECTION ( 'NONE',  ( 0.000000000000000000, 1.334402673828305746E-15, -1.000000000000000000 ) ) ;
#19749=ORIENTED_EDGE ( 'NONE', *, *, #1310, .T. ) ;
#19771=CARTESIAN_POINT ( 'NONE',  ( -69.99999999999997158, -87.33333333333338544, 3.000000000000001332 ) ) ;
#19796=CYLINDRICAL_SURFACE ( 'NONE', #9535, 2.649999999999985700 ) ;
#19800=VERTEX_POINT ( 'NONE', #16276 ) ;
#19801=EDGE_CURVE ( 'NONE', #15253, #12527, #5394, .T. ) ;
#19814=DIRECTION ( 'NONE',  ( 0.000000000000000000, -2.618450529776326854E-15, -1.000000000000000000 ) ) ;
#19816=LINE ( 'NONE', #3266, #20742 ) ;
#19878=FACE_BOUND ( 'NONE', #7001, .T. ) ;
#19896=DIRECTION ( 'NONE',  ( 1.000000000000000000, -0.000000000000000000, 0.000000000000000000 ) ) ;
#19899=VECTOR ( 'NONE', #22596, 1000.000000000000000 ) ;
#19905=ORIENTED_EDGE ( 'NONE', *, *, #21692, .T. ) ;
#19951=CARTESIAN_POINT ( 'NONE',  ( 80.00000000000001421, -59.79999999999913030, 250.0000000000000000 ) ) ;
#19952=DIRECTION ( 'NONE',  ( -3.469446951953614682E-16, 1.000000000000000000, -3.491481338843133355E-15 ) ) ;
#19974=VERTEX_POINT ( 'NONE', #20838 ) ;
#19983=VECTOR ( 'NONE', #694, 1000.000000000000000 ) ;
#19992=DIRECTION ( 'NONE',  ( -3.469446951953614682E-16, 1.000000000000000000, -3.491481338843133355E-15 ) ) ;
#19998=ORIENTED_EDGE ( 'NONE', *, *, #2696, .T. ) ;
#20001=CARTESIAN_POINT ( 'NONE',  ( -52.99999999999997158, -130.5567675943147208, 0.000000000000000000 ) ) ;
#20006=VECTOR ( 'NONE', #5246, 1000.000000000000000 ) ;
#20027=VECTOR ( 'NONE', #9467, 1000.000000000000000 ) ;
#20033=CIRCLE ( 'NONE', #3819, 2.649999999999999467 ) ;
#20038=ORIENTED_EDGE ( 'NONE', *, *, #14212, .T. ) ;
#20077=DIRECTION ( 'NONE',  ( 3.469446951953614682E-16, -1.000000000000000000, 3.483493295888648978E-15 ) ) ;
#20078=EDGE_CURVE ( 'NONE', #11951, #17193, #19476, .T. ) ;
#20101=DIRECTION ( 'NONE',  ( -1.000000000000000000, 0.000000000000000000, 0.000000000000000000 ) ) ;
#20159=DIRECTION ( 'NONE',  ( -0.000000000000000000, -0.000000000000000000, 1.000000000000000000 ) ) ;
#20187=ORIENTED_EDGE ( 'NONE', *, *, #16363, .T. ) ;
#20196=CARTESIAN_POINT ( 'NONE',  ( -52.99999999999997158, -56.80000000000005400, 2.098186183925023932E-13 ) ) ;
#20217=CARTESIAN_POINT ( 'NONE',  ( -79.99999999999995737, -138.0000000000000284, 0.000000000000000000 ) ) ;
#20240=ORIENTED_EDGE ( 'NONE', *, *, #18278, .F. ) ;
#20241=DIRECTION ( 'NONE',  ( 1.000000000000000000, 0.000000000000000000, 0.000000000000000000 ) ) ;
#20262=EDGE_CURVE ( 'NONE', #2548, #13805, #11419, .T. ) ;
#20273=CARTESIAN_POINT ( 'NONE',  ( 57.99999999999999289, 0.000000000000000000, 0.000000000000000000 ) ) ;
#20276=CARTESIAN_POINT ( 'NONE',  ( -79.99999999999995737, -62.00000000000004263, 3.000000000000000000 ) ) ;
#20290=CIRCLE ( 'NONE', #1783, 2.649999999999999467 ) ;
#20343=EDGE_LOOP ( 'NONE', ( #10992, #13696, #1501, #17372, #892, #15503, #13280, #6988, #14690, #789, #22413, #21248 ) ) ;
#20349=CARTESIAN_POINT ( 'NONE',  ( 45.00000000000002132, -52.79999999999934346, 195.0000000000002274 ) ) ;
#20362=CARTESIAN_POINT ( 'NONE',  ( 0.000000000000000000, -131.7994082814339833, 3.000000000000000000 ) ) ;
#20383=EDGE_LOOP ( 'NONE', ( #5458, #7811, #6116, #7639 ) ) ;
#20388=ORIENTED_EDGE ( 'NONE', *, *, #16574, .F. ) ;
#20394=AXIS2_PLACEMENT_3D ( 'NONE', #1616, #9356, #22021 ) ;
#20399=VECTOR ( 'NONE', #13448, 1000.000000000000000 ) ;
#20417=AXIS2_PLACEMENT_3D ( 'NONE', #15892, #23225, #19122 ) ;
#20425=DIRECTION ( 'NONE',  ( 0.000000000000000000, -2.618450529776313049E-15, -1.000000000000000000 ) ) ;
#20455=ADVANCED_FACE ( 'NONE', ( #5450 ), #8724, .F. ) ;
#20470=LINE ( 'NONE', #3799, #5540 ) ;
#20488=VERTEX_POINT ( 'NONE', #9078 ) ;
#20494=ORIENTED_EDGE ( 'NONE', *, *, #4634, .F. ) ;
#20526=ADVANCED_FACE ( 'NONE', ( #3508 ), #3610, .T. ) ;
#20530=ORIENTED_EDGE ( 'NONE', *, *, #23695, .T. ) ;
#20532=EDGE_CURVE ( 'NONE', #2917, #10831, #19816, .T. ) ;
#20543=ORIENTED_EDGE ( 'NONE', *, *, #6460, .F. ) ;
#20552=ORIENTED_EDGE ( 'NONE', *, *, #13451, .T. ) ;
#20560=DIRECTION ( 'NONE',  ( -1.000000000000000000, 0.000000000000000000, -0.000000000000000000 ) ) ;
#20569=AXIS2_PLACEMENT_3D ( 'NONE', #10528, #1667, #3354 ) ;
#20574=FACE_OUTER_BOUND ( 'NONE', #20343, .T. ) ;
#20586=DIRECTION ( 'NONE',  ( -0.000000000000000000, 1.000000000000000000, -3.469446951953613794E-15 ) ) ;
#20593=VECTOR ( 'NONE', #9112, 1000.000000000000000 ) ;
#20607=DIRECTION ( 'NONE',  ( 1.000000000000000000, -3.051161311199799893E-31, -8.144298233840332611E-17 ) ) ;
#20613=ORIENTED_EDGE ( 'NONE', *, *, #3733, .F. ) ;
#20638=DIRECTION ( 'NONE',  ( 1.000000000000000000, 0.000000000000000000, 0.000000000000000000 ) ) ;
#20657=CIRCLE ( 'NONE', #14913, 2.649999999999985700 ) ;
#20682=DIRECTION ( 'NONE',  ( 0.000000000000000000, -2.618450529776313049E-15, -1.000000000000000000 ) ) ;
#20700=ORIENTED_EDGE ( 'NONE', *, *, #12996, .F. ) ;
#20703=DIRECTION ( 'NONE',  ( 0.000000000000000000, 0.000000000000000000, -1.000000000000000000 ) ) ;
#20706=CARTESIAN_POINT ( 'NONE',  ( -59.99999999999995737, -59.79999999999975557, 74.99940828143398619 ) ) ;
#20724=ORIENTED_EDGE ( 'NONE', *, *, #9111, .T. ) ;
#20742=VECTOR ( 'NONE', #7024, 1000.000000000000000 ) ;
#20762=ADVANCED_FACE ( 'NONE', ( #17841 ), #14127, .T. ) ;
#20763=AXIS2_PLACEMENT_3D ( 'NONE', #10738, #3330, #21699 ) ;
#20781=AXIS2_PLACEMENT_3D ( 'NONE', #14527, #18144, #14649 ) ;
#20809=VECTOR ( 'NONE', #974, 1000.000000000000000 ) ;
#20838=CARTESIAN_POINT ( 'NONE',  ( 50.00000000000000000, -59.79999999999974847, 74.99940828143402882 ) ) ;
#20864=DIRECTION ( 'NONE',  ( -3.051161311199799893E-31, -1.000000000000000000, 0.000000000000000000 ) ) ;
#20883=ORIENTED_EDGE ( 'NONE', *, *, #8782, .T. ) ;
#20903=FACE_OUTER_BOUND ( 'NONE', #14066, .T. ) ;
#20909=LINE ( 'NONE', #11772, #8677 ) ;
#20911=VERTEX_POINT ( 'NONE', #9023 ) ;
#20913=DIRECTION ( 'NONE',  ( 0.000000000000000000, -2.618450529776326854E-15, -1.000000000000000000 ) ) ;
#20914=ORIENTED_EDGE ( 'NONE', *, *, #12148, .F. ) ;
#20922=EDGE_LOOP ( 'NONE', ( #7622, #1723, #1193, #5171 ) ) ;
#20931=ORIENTED_EDGE ( 'NONE', *, *, #215, .F. ) ;
#20941=DIRECTION ( 'NONE',  ( 0.000000000000000000, -2.618450529776313049E-15, -1.000000000000000000 ) ) ;
#20961=FACE_OUTER_BOUND ( 'NONE', #22929, .T. ) ;
#20983=ADVANCED_FACE ( 'NONE', ( #22403 ), #18898, .F. ) ;
#20994=ORIENTED_EDGE ( 'NONE', *, *, #20532, .T. ) ;
#21002=ORIENTED_EDGE ( 'NONE', *, *, #10358, .F. ) ;
#21012=CARTESIAN_POINT ( 'NONE',  ( -44.99999999999995026, -56.79999999999968452, 105.0000000000002132 ) ) ;
#21013=ADVANCED_FACE ( 'NONE', ( #2591 ), #2109, .F. ) ;
#21019=VECTOR ( 'NONE', #2986, 1000.000000000000000 ) ;
#21038=VECTOR ( 'NONE', #7728, 1000.000000000000000 ) ;
#21045=ORIENTED_EDGE ( 'NONE', *, *, #4999, .F. ) ;
#21048=VECTOR ( 'NONE', #18289, 1000.000000000000000 ) ;
#21064=DIRECTION ( 'NONE',  ( 0.000000000000000000, 1.334402673828305746E-15, -1.000000000000000000 ) ) ;
#21070=FACE_OUTER_BOUND ( 'NONE', #1348, .T. ) ;
#21116=CARTESIAN_POINT ( 'NONE',  ( 80.00000000000000000, -61.99999999999998579, 3.000000000000000000 ) ) ;
#21119=AXIS2_PLACEMENT_3D ( 'NONE', #48, #21656, #3523 ) ;
#21123=ORIENTED_EDGE ( 'NONE', *, *, #16358, .F. ) ;
#21139=VERTEX_POINT ( 'NONE', #6106 ) ;
#21161=ORIENTED_EDGE ( 'NONE', *, *, #904, .F. ) ;
#21171=AXIS2_PLACEMENT_3D ( 'NONE', #7765, #269, #20913 ) ;
#21172=VECTOR ( 'NONE', #17371, 1000.000000000000000 ) ;
#21187=PLANE ( 'NONE',  #20417 ) ;
#21199=DIRECTION ( 'NONE',  ( -0.000000000000000000, 1.000000000000000000, -3.469446951953613794E-15 ) ) ;
#21227=DIRECTION ( 'NONE',  ( 1.000000000000000000, 0.000000000000000000, 0.000000000000000000 ) ) ;
#21232=LINE ( 'NONE', #1177, #9414 ) ;
#21234=CARTESIAN_POINT ( 'NONE',  ( 52.00000000000000711, -56.79999999999974847, 75.17098115668785852 ) ) ;
#21248=ORIENTED_EDGE ( 'NONE', *, *, #19013, .F. ) ;
#21281=EDGE_CURVE ( 'NONE', #16291, #5557, #7052, .T. ) ;
#21300=ADVANCED_FACE ( 'NONE', ( #14683 ), #21889, .F. ) ;
#21319=CYLINDRICAL_SURFACE ( 'NONE', #16125, 2.649999999999985700 ) ;
#21321=ORIENTED_EDGE ( 'NONE', *, *, #15908, .F. ) ;
#21439=CARTESIAN_POINT ( 'NONE',  ( 67.35000000000002274, -112.6666666666666714, 0.000000000000000000 ) ) ;
#21440=EDGE_CURVE ( 'NONE', #1247, #9060, #19568, .T. ) ;
#21477=EDGE_LOOP ( 'NONE', ( #1214, #1854, #7194, #20931 ) ) ;
#21511=AXIS2_PLACEMENT_3D ( 'NONE', #17165, #21708, #2423 ) ;
#21512=CARTESIAN_POINT ( 'NONE',  ( 57.99999999999997868, -62.00000000000001421, 5.199999999999997513 ) ) ;
#21520=DIRECTION ( 'NONE',  ( -8.144298233840332611E-17, 0.000000000000000000, -1.000000000000000000 ) ) ;
#21531=DIRECTION ( 'NONE',  ( -0.000000000000000000, -0.000000000000000000, 1.000000000000000000 ) ) ;
#21539=ORIENTED_EDGE ( 'NONE', *, *, #18331, .F. ) ;
#21550=DIRECTION ( 'NONE',  ( 0.000000000000000000, -2.618450529776326854E-15, -1.000000000000000000 ) ) ;
#21566=CARTESIAN_POINT ( 'NONE',  ( 45.00000000000002132, -59.79999999999933635, 195.0000000000002558 ) ) ;
#21578=LINE ( 'NONE', #6610, #16031 ) ;
#21591=CARTESIAN_POINT ( 'NONE',  ( -72.64999999999994884, -112.6666666666667140, 3.000000000000001332 ) ) ;
#21595=EDGE_LOOP ( 'NONE', ( #23248, #3226 ) ) ;
#21605=DIRECTION ( 'NONE',  ( -0.000000000000000000, 1.000000000000000000, -3.469446951953613794E-15 ) ) ;
#21614=STYLED_ITEM ( 'NONE', ( #4957 ), #5011 ) ;
#21626=ORIENTED_EDGE ( 'NONE', *, *, #3733, .T. ) ;
#21627=EDGE_CURVE ( 'NONE', #10418, #3759, #7285, .T. ) ;
#21632=VECTOR ( 'NONE', #209, 1000.000000000000000 ) ;
#21651=LINE ( 'NONE', #9089, #4243 ) ;
#21653=DIRECTION ( 'NONE',  ( 1.000000000000000000, -3.051161311199799893E-31, -8.144298233840332611E-17 ) ) ;
#21656=DIRECTION ( 'NONE',  ( -1.000000000000000000, -5.478074134663600261E-16, 0.000000000000000000 ) ) ;
#21663=CARTESIAN_POINT ( 'NONE',  ( 80.00000000000004263, -137.9999999999999716, 3.000000000000000000 ) ) ;
#21670=CARTESIAN_POINT ( 'NONE',  ( -49.99999999999997158, -138.3994082814338071, -3.599999999999746070 ) ) ;
#21692=EDGE_CURVE ( 'NONE', #18517, #19974, #9083, .T. ) ;
#21699=DIRECTION ( 'NONE',  ( 0.000000000000000000, 0.000000000000000000, -1.000000000000000000 ) ) ;
#21708=DIRECTION ( 'NONE',  ( -1.000000000000000000, -3.469446951953612710E-16, 5.618537574014070918E-17 ) ) ;
#21710=ORIENTED_EDGE ( 'NONE', *, *, #19409, .T. ) ;
#21716=FACE_OUTER_BOUND ( 'NONE', #21477, .T. ) ;
#21740=CARTESIAN_POINT ( 'NONE',  ( -56.99999999999995737, -62.00000000000001421, 5.199999999999997513 ) ) ;
#21744=EDGE_CURVE ( 'NONE', #7697, #4863, #21879, .T. ) ;
#21748=ORIENTED_EDGE ( 'NONE', *, *, #15881, .T. ) ;
#21777=VECTOR ( 'NONE', #15967, 1000.000000000000000 ) ;
#21779=VECTOR ( 'NONE', #15613, 1000.000000000000000 ) ;
#21807=PLANE ( 'NONE',  #17504 ) ;
#21852=ORIENTED_EDGE ( 'NONE', *, *, #15980, .T. ) ;
#21859=DIRECTION ( 'NONE',  ( -1.000000000000000000, -0.000000000000000000, -0.000000000000000000 ) ) ;
#21873=VECTOR ( 'NONE', #12465, 1000.000000000000000 ) ;
#21879=CIRCLE ( 'NONE', #5311, 2.649999999999985700 ) ;
#21889=CYLINDRICAL_SURFACE ( 'NONE', #20394, 2.200000000000028155 ) ;
#21902=DIRECTION ( 'NONE',  ( 5.618537574013950123E-17, 3.483493295888648978E-15, 1.000000000000000000 ) ) ;
#21915=AXIS2_PLACEMENT_3D ( 'NONE', #21512, #23675, #1589 ) ;
#21944=CARTESIAN_POINT ( 'NONE',  ( -79.99999999999995737, -62.00000000000007816, -3.122502256758252770E-14 ) ) ;
#21948=EDGE_LOOP ( 'NONE', ( #19435, #16482, #22132, #17514 ) ) ;
#21967=VECTOR ( 'NONE', #633, 1000.000000000000000 ) ;
#21976=AXIS2_PLACEMENT_3D ( 'NONE', #10176, #17419, #18967 ) ;
#22004=DIRECTION ( 'NONE',  ( 0.000000000000000000, -2.618450529776326854E-15, -1.000000000000000000 ) ) ;
#22011=ORIENTED_EDGE ( 'NONE', *, *, #16828, .F. ) ;
#22021=DIRECTION ( 'NONE',  ( 0.000000000000000000, 1.000000000000000000, -3.548298019043423769E-15 ) ) ;
#22027=ORIENTED_EDGE ( 'NONE', *, *, #849, .F. ) ;
#22056=FACE_OUTER_BOUND ( 'NONE', #14554, .T. ) ;
#22072=PLANE ( 'NONE',  #13477 ) ;
#22132=ORIENTED_EDGE ( 'NONE', *, *, #9009, .F. ) ;
#22162=ORIENTED_EDGE ( 'NONE', *, *, #1212, .T. ) ;
#22167=EDGE_CURVE ( 'NONE', #16172, #11184, #4555, .T. ) ;
#22188=ORIENTED_EDGE ( 'NONE', *, *, #21692, .F. ) ;
#22199=ORIENTED_EDGE ( 'NONE', *, *, #12148, .T. ) ;
#22217=ORIENTED_EDGE ( 'NONE', *, *, #21627, .F. ) ;
#22229=ORIENTED_EDGE ( 'NONE', *, *, #9906, .T. ) ;
#22231=CARTESIAN_POINT ( 'NONE',  ( -44.99999999999995026, -59.79999999999967741, 107.6500000000002331 ) ) ;
#22261=VERTEX_POINT ( 'NONE', #8279 ) ;
#22278=AXIS2_PLACEMENT_3D ( 'NONE', #1374, #21199, #8761 ) ;
#22280=AXIS2_PLACEMENT_3D ( 'NONE', #6118, #13403, #7688 ) ;
#22299=ADVANCED_FACE ( 'NONE', ( #21070, #11447, #16988, #668, #444 ), #7795, .T. ) ;
#22307=ADVANCED_FACE ( 'NONE', ( #19254 ), #18894, .F. ) ;
#22330=( NAMED_UNIT ( * ) SI_UNIT ( $, .STERADIAN. ) SOLID_ANGLE_UNIT ( ) );
#22349=ORIENTED_EDGE ( 'NONE', *, *, #12694, .F. ) ;
#22365=FACE_OUTER_BOUND ( 'NONE', #23235, .T. ) ;
#22367=CARTESIAN_POINT ( 'NONE',  ( 80.00000000000001421, -59.79999999999998295, 5.199999999999996625 ) ) ;
#22383=DIRECTION ( 'NONE',  ( 0.000000000000000000, 0.000000000000000000, -1.000000000000000000 ) ) ;
#22403=FACE_OUTER_BOUND ( 'NONE', #11937, .T. ) ;
#22412=ADVANCED_FACE ( 'NONE', ( #4764 ), #1008, .F. ) ;
#22413=ORIENTED_EDGE ( 'NONE', *, *, #4353, .F. ) ;
#22453=DIRECTION ( 'NONE',  ( 0.000000000000000000, -2.618450529776313049E-15, -1.000000000000000000 ) ) ;
#22495=CARTESIAN_POINT ( 'NONE',  ( 45.00000000000004974, -59.79999999999964899, 105.0000000000002274 ) ) ;
#22509=CARTESIAN_POINT ( 'NONE',  ( -44.99999999999995026, -56.79999999999969162, 102.3500000000002217 ) ) ;
#22544=DIRECTION ( 'NONE',  ( 1.000000000000000000, 0.000000000000000000, 0.000000000000000000 ) ) ;
#22547=VECTOR ( 'NONE', #11894, 1000.000000000000000 ) ;
#22572=FACE_OUTER_BOUND ( 'NONE', #14651, .T. ) ;
#22596=DIRECTION ( 'NONE',  ( -1.000000000000000000, -3.469446951953617640E-16, -8.673617379884035472E-17 ) ) ;
#22627=CARTESIAN_POINT ( 'NONE',  ( -52.99999999999997158, -62.00000000000001421, 5.199999999999997513 ) ) ;
#22628=VERTEX_POINT ( 'NONE', #9713 ) ;
#22634=DIRECTION ( 'NONE',  ( 0.000000000000000000, -2.618450529776313049E-15, -1.000000000000000000 ) ) ;
#22649=CYLINDRICAL_SURFACE ( 'NONE', #19209, 2.200000000000028155 ) ;
#22656=ORIENTED_EDGE ( 'NONE', *, *, #19583, .T. ) ;
#22680=AXIS2_PLACEMENT_3D ( 'NONE', #21566, #5031, #10600 ) ;
#22745=EDGE_CURVE ( 'NONE', #5068, #11184, #281, .T. ) ;
#22762=CARTESIAN_POINT ( 'NONE',  ( 60.00000000000000000, -137.1994082814340743, -2.400000000000046096 ) ) ;
#22768=CARTESIAN_POINT ( 'NONE',  ( 57.99999999999999289, 0.000000000000000000, 0.000000000000000000 ) ) ;
#22792=DIRECTION ( 'NONE',  ( -0.000000000000000000, -0.000000000000000000, 1.000000000000000000 ) ) ;
#22814=ORIENTED_EDGE ( 'NONE', *, *, #8713, .T. ) ;
#22824=EDGE_CURVE ( 'NONE', #16291, #1461, #3491, .T. ) ;
#22858=CARTESIAN_POINT ( 'NONE',  ( 80.00000000000001421, -59.79999999999998295, 5.199999999999996625 ) ) ;
#22925=AXIS2_PLACEMENT_3D ( 'NONE', #23369, #17825, #18181 ) ;
#22929=EDGE_LOOP ( 'NONE', ( #6772, #23263, #22814, #1939 ) ) ;
#22952=ADVANCED_FACE ( 'NONE', ( #14738 ), #22072, .T. ) ;
#22971=LINE ( 'NONE', #12523, #2654 ) ;
#22972=CARTESIAN_POINT ( 'NONE',  ( 72.64999999999999147, -87.33333333333332860, 0.000000000000000000 ) ) ;
#22974=DIRECTION ( 'NONE',  ( -3.469446951953614682E-16, 1.000000000000000000, -3.483493295888648978E-15 ) ) ;
#22982=DIRECTION ( 'NONE',  ( -0.000000000000000000, 1.000000000000000000, -3.469446951953613794E-15 ) ) ;
#23011=CARTESIAN_POINT ( 'NONE',  ( 45.00000000000004974, -59.79999999999964189, 107.6500000000002331 ) ) ;
#23022=CARTESIAN_POINT ( 'NONE',  ( -44.99999999999997868, -52.79999999999936477, 197.6500000000001478 ) ) ;
#23038=VERTEX_POINT ( 'NONE', #5537 ) ;
#23041=ADVANCED_FACE ( 'NONE', ( #12100 ), #15807, .F. ) ;
#23050=ORIENTED_EDGE ( 'NONE', *, *, #15634, .T. ) ;
#23054=SURFACE_SIDE_STYLE ('',( #2776 ) ) ;
#23072=ORIENTED_EDGE ( 'NONE', *, *, #19625, .T. ) ;
#23090=VECTOR ( 'NONE', #19992, 1000.000000000000000 ) ;
#23102=ORIENTED_EDGE ( 'NONE', *, *, #17663, .T. ) ;
#23132=AXIS2_PLACEMENT_3D ( 'NONE', #19771, #10630, #7987 ) ;
#23133=CIRCLE ( 'NONE', #2698, 2.649999999999985700 ) ;
#23155=CARTESIAN_POINT ( 'NONE',  ( -44.99999999999995026, -52.79999999999967741, 105.0000000000001990 ) ) ;
#23161=DIRECTION ( 'NONE',  ( 0.000000000000000000, -2.618450529776326854E-15, -1.000000000000000000 ) ) ;
#23175=LINE ( 'NONE', #6755, #17726 ) ;
#23186=( NAMED_UNIT ( * ) PLANE_ANGLE_UNIT ( ) SI_UNIT ( $, .RADIAN. ) );
#23190=VERTEX_POINT ( 'NONE', #21234 ) ;
#23225=DIRECTION ( 'NONE',  ( 1.000000000000000000, 0.000000000000000000, 0.000000000000000000 ) ) ;
#23226=DIRECTION ( 'NONE',  ( 1.000000000000000000, 0.000000000000000000, 0.000000000000000000 ) ) ;
#23235=EDGE_LOOP ( 'NONE', ( #1448, #20388, #16230, #21748 ) ) ;
#23248=ORIENTED_EDGE ( 'NONE', *, *, #9923, .F. ) ;
#23261=ADVANCED_FACE ( 'NONE', ( #18080 ), #5157, .F. ) ;
#23263=ORIENTED_EDGE ( 'NONE', *, *, #4062, .F. ) ;
#23276=ORIENTED_EDGE ( 'NONE', *, *, #13674, .T. ) ;
#23292=DIRECTION ( 'NONE',  ( -3.051161311199799893E-31, -1.000000000000000000, 0.000000000000000000 ) ) ;
#23312=VERTEX_POINT ( 'NONE', #1644 ) ;
#23339=DIRECTION ( 'NONE',  ( -0.000000000000000000, -0.000000000000000000, 1.000000000000000000 ) ) ;
#23360=AXIS2_PLACEMENT_3D ( 'NONE', #21740, #122, #5202 ) ;
#23369=CARTESIAN_POINT ( 'NONE',  ( 80.00000000000000000, -62.00000000000001421, 5.199999999999997513 ) ) ;
#23374=ORIENTED_EDGE ( 'NONE', *, *, #18278, .T. ) ;
#23407=DIRECTION ( 'NONE',  ( 0.000000000000000000, 0.000000000000000000, -1.000000000000000000 ) ) ;
#23411=DIRECTION ( 'NONE',  ( 5.758888509154132365E-17, 0.7071067811865489050, 0.7071067811865462405 ) ) ;
#23445=ORIENTED_EDGE ( 'NONE', *, *, #937, .F. ) ;
#23454=AXIS2_PLACEMENT_3D ( 'NONE', #13657, #9649, #13184 ) ;
#23502=CIRCLE ( 'NONE', #4219, 2.649999999999999467 ) ;
#23514=CARTESIAN_POINT ( 'NONE',  ( 70.00000000000000000, -87.33333333333332860, 3.000000000000000000 ) ) ;
#23519=VERTEX_POINT ( 'NONE', #20706 ) ;
#23559=ORIENTED_EDGE ( 'NONE', *, *, #6954, .F. ) ;
#23561=ORIENTED_EDGE ( 'NONE', *, *, #7344, .F. ) ;
#23563=ORIENTED_EDGE ( 'NONE', *, *, #12157, .T. ) ;
#23579=EDGE_CURVE ( 'NONE', #9060, #12933, #15547, .T. ) ;
#23668=DIRECTION ( 'NONE',  ( -1.000000000000000000, -0.000000000000000000, -0.000000000000000000 ) ) ;
#23675=DIRECTION ( 'NONE',  ( -1.000000000000000000, 0.000000000000000000, -0.000000000000000000 ) ) ;
#23695=EDGE_CURVE ( 'NONE', #326, #19241, #10711, .T. ) ;
#23724=LINE ( 'NONE', #9264, #21048 ) ;
#23731=AXIS2_PLACEMENT_3D ( 'NONE', #18940, #240, #13314 ) ;
#23733=CARTESIAN_POINT ( 'NONE',  ( 60.00000000000000000, -61.99999999999999289, 3.000000000000000000 ) ) ;
#23747=VECTOR ( 'NONE', #21902, 1000.000000000000000 ) ;
#23781=EDGE_CURVE ( 'NONE', #506, #5068, #743, .T. ) ;
#23907=COLOUR_RGB('Sky Blue',0.24,0.69,0.87);
#23908=FILL_AREA_STYLE_COLOUR('',#23907);
#23909=FILL_AREA_STYLE('',(#23908));
#23910=SURFACE_STYLE_FILL_AREA(#23909);
#23911=SURFACE_SIDE_STYLE('',(#23910));
#23912=SURFACE_STYLE_USAGE(.BOTH.,#23911);
#23913=PRESENTATION_STYLE_ASSIGNMENT((#23912));
ENDSEC;
END-ISO-10303-21;
